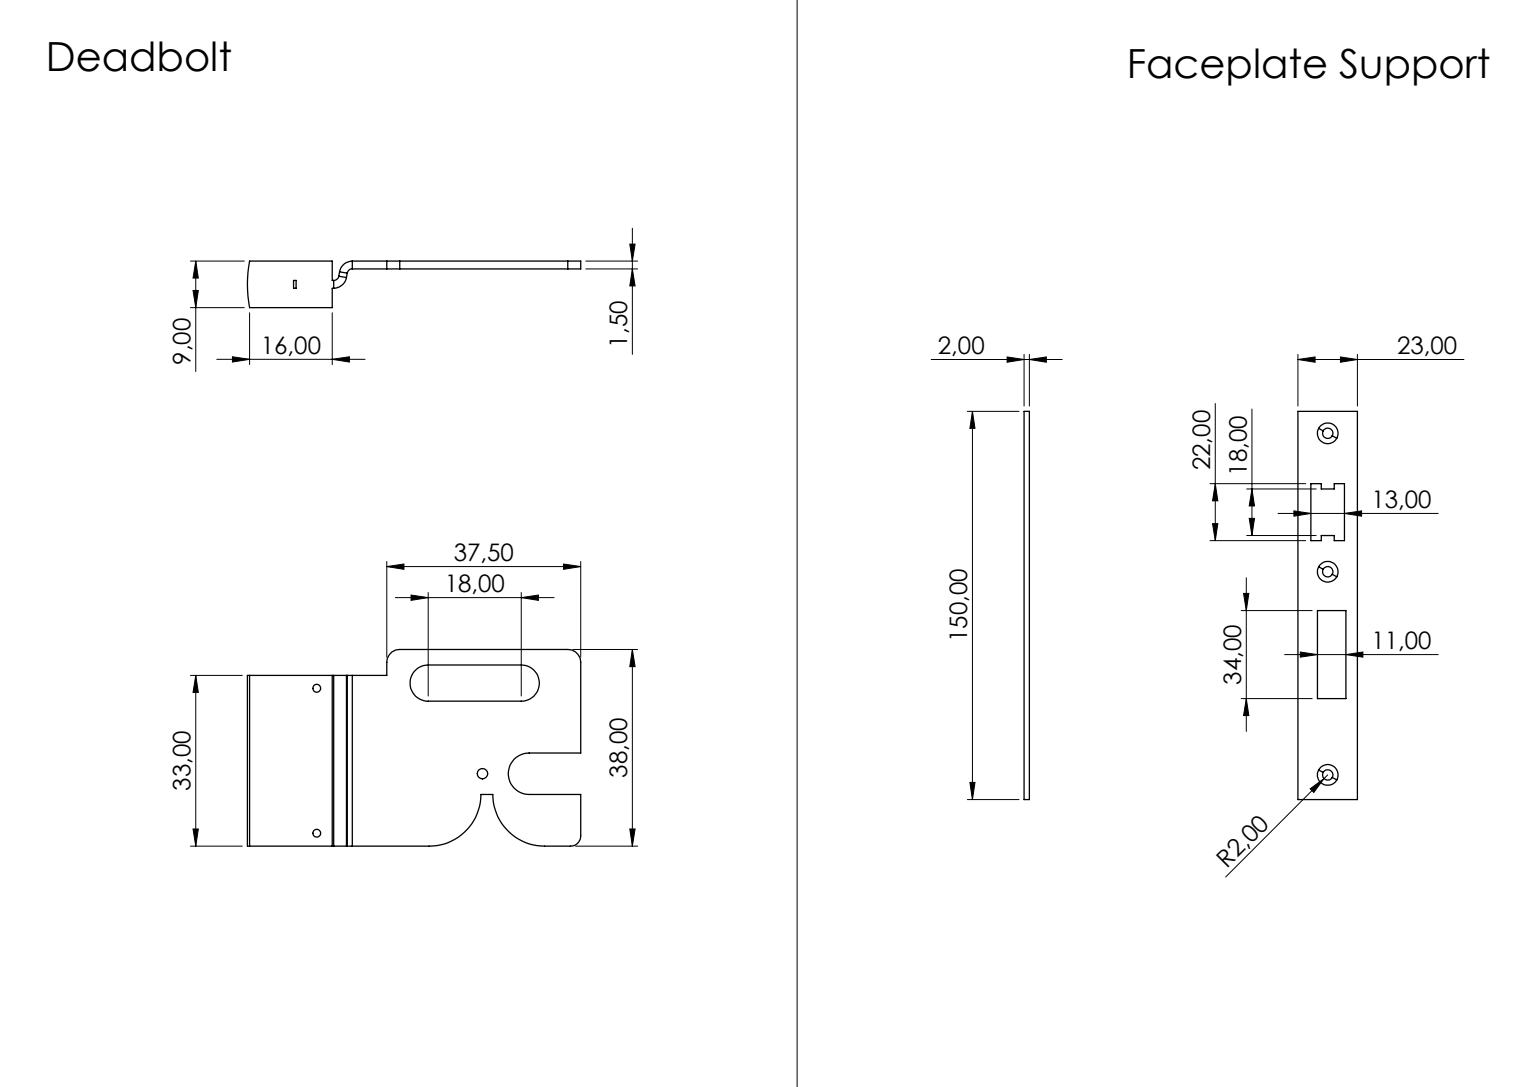
ISO-10303-21;
HEADER;
FILE_DESCRIPTION (('STEP AP214'),
    '1' );
FILE_NAME ('Faceplate Support.step',
    '2026-10-06T13:23:30',
    ( '' ),
    ( '' ),
    'SwSTEP 2.0',
    'SolidWorks 2020',
    '' );
FILE_SCHEMA (( 'AUTOMOTIVE_DESIGN' ));
ENDSEC;

DATA;
#73=VERTEX_POINT ( 'NONE', #5299 ) ;
#76=VERTEX_POINT ( 'NONE', #12547 ) ;
#94=VECTOR ( 'NONE', #6253, 1000.000000000000000 ) ;
#132=DIRECTION ( 'NONE',  ( 1.000000000000000000, 0.000000000000000000, 0.000000000000000000 ) ) ;
#135=DIRECTION ( 'NONE',  ( 1.000000000000000000, 2.602084704489999637E-17, 0.000000000000000000 ) ) ;
#145=FACE_BOUND ( 'NONE', #10019, .T. ) ;
#180=CARTESIAN_POINT ( 'NONE',  ( -33.42928932190000069, 66.02782287919998794, -146.7500980969999773 ) ) ;
#183=EDGE_LOOP ( 'NONE', ( #12514, #3187, #13299, #6261 ) ) ;
#184=EDGE_LOOP ( 'NONE', ( #18556, #23230 ) ) ;
#210=ADVANCED_FACE ( 'NONE', ( #13249 ), #13024, .F. ) ;
#292=LINE ( 'NONE', #7531, #4006 ) ;
#309=EDGE_LOOP ( 'NONE', ( #20160, #3924, #21001, #22212 ) ) ;
#317=CONICAL_SURFACE ( 'NONE', #15128, 1.999999999999992450, 0.7853981633970000820 ) ;
#385=FILL_AREA_STYLE_COLOUR ( '', #1433 ) ;
#392=LINE ( 'NONE', #16802, #3859 ) ;
#419=EDGE_LOOP ( 'NONE', ( #6689, #18751, #11885, #12680 ) ) ;
#431=ORIENTED_EDGE ( 'NONE', *, *, #17551, .T. ) ;
#453=ORIENTED_EDGE ( 'NONE', *, *, #12083, .T. ) ;
#485=PRESENTATION_STYLE_ASSIGNMENT (( #16769 ) ) ;
#517=DIRECTION ( 'NONE',  ( 0.000000000000000000, 0.000000000000000000, 1.000000000000000000 ) ) ;
#555=DIRECTION ( 'NONE',  ( -1.000000000000000000, 0.000000000000000000, 1.701177084980000217E-20 ) ) ;
#577=DIRECTION ( 'NONE',  ( 0.000000000000000000, -1.000000000000000000, 0.000000000000000000 ) ) ;
#623=PLANE ( 'NONE',  #6012 ) ;
#626=CARTESIAN_POINT ( 'NONE',  ( -32.50000000000000000, 27.00000000000000000, -141.5552959529999839 ) ) ;
#725=DIRECTION ( 'NONE',  ( 0.000000000000000000, 1.000000000000000000, 0.000000000000000000 ) ) ;
#777=VERTEX_POINT ( 'NONE', #13933 ) ;
#800=ORIENTED_EDGE ( 'NONE', *, *, #6653, .T. ) ;
#823=VECTOR ( 'NONE', #20074, 1000.000000000000000 ) ;
#843=CARTESIAN_POINT ( 'NONE',  ( -34.50000000000000000, -35.00000000000000000, -151.0552959529999839 ) ) ;
#845=VECTOR ( 'NONE', #2349, 1000.000000000000000 ) ;
#924=PLANE ( 'NONE',  #10610 ) ;
#925=CARTESIAN_POINT ( 'NONE',  ( -32.50000000000000000, 76.00000000000000000, -132.5552959530000123 ) ) ;
#927=CARTESIAN_POINT ( 'NONE',  ( -33.50000000000000000, -35.00000000000000000, -151.0552959529999839 ) ) ;
#941=VERTEX_POINT ( 'NONE', #11143 ) ;
#947=VERTEX_POINT ( 'NONE', #8804 ) ;
#969=DIRECTION ( 'NONE',  ( -1.000000000000000000, -2.602084704489999637E-17, 1.701177084830000066E-20 ) ) ;
#971=LINE ( 'NONE', #21197, #17113 ) ;
#1010=VECTOR ( 'NONE', #18945, 1000.000000000000000 ) ;
#1022=FACE_OUTER_BOUND ( 'NONE', #1478, .T. ) ;
#1026=LINE ( 'NONE', #6599, #12411 ) ;
#1069=VERTEX_POINT ( 'NONE', #925 ) ;
#1108=FACE_OUTER_BOUND ( 'NONE', #16737, .T. ) ;
#1156=VECTOR ( 'NONE', #20344, 1000.000000000000000 ) ;
#1161=DIRECTION ( 'NONE',  ( 1.000000000000000000, 0.000000000000000000, 0.000000000000000000 ) ) ;
#1195=DIRECTION ( 'NONE',  ( 1.000000000000000000, 2.004714280773594901E-17, -1.095180403012019938E-17 ) ) ;
#1238=AXIS2_PLACEMENT_3D ( 'NONE', #1926, #9145, #135 ) ;
#1262=DIRECTION ( 'NONE',  ( 0.000000000000000000, 0.000000000000000000, 1.000000000000000000 ) ) ;
#1350=LINE ( 'NONE', #10594, #19286 ) ;
#1398=EDGE_CURVE ( 'NONE', #23370, #2980, #10145, .T. ) ;
#1419=EDGE_CURVE ( 'NONE', #22886, #9252, #5700, .T. ) ;
#1422=VERTEX_POINT ( 'NONE', #4812 ) ;
#1433=COLOUR_RGB ( '', 0.31764706, 0.68627451, 0.89019608) ;
#1467=ADVANCED_FACE ( 'NONE', ( #15641 ), #8127, .F. ) ;
#1478=EDGE_LOOP ( 'NONE', ( #5603, #15343, #800, #15418 ) ) ;
#1527=VECTOR ( 'NONE', #2984, 1000.000000000000000 ) ;
#1629=PRODUCT ( 'Faceplate Support', 'Faceplate Support', '', ( #5675 ) ) ;
#1638=EDGE_LOOP ( 'NONE', ( #18762, #8978 ) ) ;
#1718=EDGE_CURVE ( 'NONE', #3899, #19035, #971, .T. ) ;
#1720=( LENGTH_UNIT ( ) NAMED_UNIT ( * ) SI_UNIT ( .MILLI., .METRE. ) );
#1770=EDGE_CURVE ( 'NONE', #4685, #18991, #9262, .T. ) ;
#1772=ORIENTED_EDGE ( 'NONE', *, *, #22316, .F. ) ;
#1774=ORIENTED_EDGE ( 'NONE', *, *, #4121, .F. ) ;
#1780=AXIS2_PLACEMENT_3D ( 'NONE', #5327, #3659, #9112 ) ;
#1819=ORIENTED_EDGE ( 'NONE', *, *, #16781, .T. ) ;
#1849=LINE ( 'NONE', #20040, #1010 ) ;
#1926=CARTESIAN_POINT ( 'NONE',  ( -32.50000000000000000, 48.00000000000000000, -146.5552959529999839 ) ) ;
#1931=DIRECTION ( 'NONE',  ( 0.000000000000000000, 1.000000000000000000, 0.000000000000000000 ) ) ;
#1948=LINE ( 'NONE', #3834, #4457 ) ;
#1951=DIRECTION ( 'NONE',  ( 1.000000000000000000, 2.004714280773594901E-17, -1.095180403012019938E-17 ) ) ;
#1984=ORIENTED_EDGE ( 'NONE', *, *, #6937, .F. ) ;
#2041=FACE_OUTER_BOUND ( 'NONE', #13396, .T. ) ;
#2052=CARTESIAN_POINT ( 'NONE',  ( -32.50000000000000000, 14.00000000000000000, -144.0552959529999839 ) ) ;
#2076=ORIENTED_EDGE ( 'NONE', *, *, #19643, .T. ) ;
#2094=ORIENTED_EDGE ( 'NONE', *, *, #16952, .F. ) ;
#2109=EDGE_CURVE ( 'NONE', #16248, #22948, #20352, .T. ) ;
#2111=VERTEX_POINT ( 'NONE', #11280 ) ;
#2132=ORIENTED_EDGE ( 'NONE', *, *, #13601, .T. ) ;
#2147=CARTESIAN_POINT ( 'NONE',  ( -34.50000000000000000, -1.000000000000000000, -145.5552959529999839 ) ) ;
#2158=DIRECTION ( 'NONE',  ( -1.000000000000000000, 0.000000000000000000, 0.000000000000000000 ) ) ;
#2182=PLANE ( 'NONE',  #20224 ) ;
#2191=EDGE_CURVE ( 'NONE', #4452, #11004, #2968, .T. ) ;
#2227=LINE ( 'NONE', #7560, #3466 ) ;
#2235=ORIENTED_EDGE ( 'NONE', *, *, #2191, .T. ) ;
#2272=FILL_AREA_STYLE_COLOUR ( '', #5063 ) ;
#2282=CARTESIAN_POINT ( 'NONE',  ( -32.50000000000000000, 48.00000000000000000, -139.5552959529999839 ) ) ;
#2311=VECTOR ( 'NONE', #4811, 1000.000000000000000 ) ;
#2349=DIRECTION ( 'NONE',  ( 0.000000000000000000, 0.000000000000000000, -1.000000000000000000 ) ) ;
#2386=CARTESIAN_POINT ( 'NONE',  ( -33.50000000000000000, 28.00000000000000000, -141.5552959529999839 ) ) ;
#2403=CARTESIAN_POINT ( 'NONE',  ( -32.50000000000000000, -1.000000000000000000, -151.0552959529999839 ) ) ;
#2432=EDGE_CURVE ( 'NONE', #18991, #13154, #12548, .T. ) ;
#2445=ORIENTED_EDGE ( 'NONE', *, *, #3029, .F. ) ;
#2460=PLANE ( 'NONE',  #7430 ) ;
#2478=DIRECTION ( 'NONE',  ( 0.000000000000000000, 1.000000000000000000, 0.000000000000000000 ) ) ;
#2576=CARTESIAN_POINT ( 'NONE',  ( -34.50000000000000000, -64.50000000000000000, -144.0552959529999839 ) ) ;
#2654=VECTOR ( 'NONE', #22857, 1000.000000000000000 ) ;
#2688=VECTOR ( 'NONE', #6527, 1000.000000000000000 ) ;
#2728=LINE ( 'NONE', #2835, #13984 ) ;
#2789=VERTEX_POINT ( 'NONE', #3495 ) ;
#2796=CARTESIAN_POINT ( 'NONE',  ( -32.50000000000000000, 48.00000000000000000, -148.5552959529999839 ) ) ;
#2797=DIRECTION ( 'NONE',  ( 1.000000000000000000, 2.602084704489999637E-17, -1.701177084830000066E-20 ) ) ;
#2835=CARTESIAN_POINT ( 'NONE',  ( -33.42928932190000069, 15.47217712079999963, -141.3604938089999905 ) ) ;
#2925=EDGE_LOOP ( 'NONE', ( #21956, #13989, #16727, #2445 ) ) ;
#2940=DIRECTION ( 'NONE',  ( 1.000000000000000000, 2.602084704489999637E-17, 0.000000000000000000 ) ) ;
#2955=CARTESIAN_POINT ( 'NONE',  ( -32.50000000000000000, -35.00000000000000000, -145.5552959529999839 ) ) ;
#2968=LINE ( 'NONE', #15450, #2688 ) ;
#2974=CARTESIAN_POINT ( 'NONE',  ( -34.50000000000000000, 67.50000000000000000, -144.0552959529999839 ) ) ;
#2980=VERTEX_POINT ( 'NONE', #4420 ) ;
#2984=DIRECTION ( 'NONE',  ( 0.000000000000000000, 1.000000000000000000, 0.000000000000000000 ) ) ;
#3029=EDGE_CURVE ( 'NONE', #1422, #22304, #7634, .T. ) ;
#3073=DIRECTION ( 'NONE',  ( 0.000000000000000000, 1.000000000000000000, 0.000000000000000000 ) ) ;
#3106=DIRECTION ( 'NONE',  ( 0.000000000000000000, 1.000000000000000000, 0.000000000000000000 ) ) ;
#3182=ORIENTED_EDGE ( 'NONE', *, *, #7620, .T. ) ;
#3187=ORIENTED_EDGE ( 'NONE', *, *, #20709, .F. ) ;
#3241=CARTESIAN_POINT ( 'NONE',  ( -32.50000000000000000, 48.00000000000000000, -146.5552959529999839 ) ) ;
#3284=VERTEX_POINT ( 'NONE', #20004 ) ;
#3338=VECTOR ( 'NONE', #7879, 1000.000000000000000 ) ;
#3382=DIRECTION ( 'NONE',  ( 0.000000000000000000, 1.000000000000000000, 0.000000000000000000 ) ) ;
#3388=ORIENTED_EDGE ( 'NONE', *, *, #3978, .T. ) ;
#3415=VECTOR ( 'NONE', #7837, 1000.000000000000000 ) ;
#3440=EDGE_CURVE ( 'NONE', #7907, #16321, #14757, .T. ) ;
#3466=VECTOR ( 'NONE', #22093, 1000.000000000000000 ) ;
#3482=DIRECTION ( 'NONE',  ( 0.000000000000000000, -0.4794255386042033384, -0.8775825618903726477 ) ) ;
#3495=CARTESIAN_POINT ( 'NONE',  ( -32.50000000000000000, 26.00000000000000000, -137.5552959530000123 ) ) ;
#3509=LINE ( 'NONE', #23142, #12900 ) ;
#3521=ORIENTED_EDGE ( 'NONE', *, *, #20709, .T. ) ;
#3536=( GEOMETRIC_REPRESENTATION_CONTEXT ( 3 ) GLOBAL_UNCERTAINTY_ASSIGNED_CONTEXT ( ( #12778 ) ) GLOBAL_UNIT_ASSIGNED_CONTEXT ( ( #1720, #9723, #18552 ) ) REPRESENTATION_CONTEXT ( 'NONE', 'WORKASPACE' ) );
#3538=VECTOR ( 'NONE', #15894, 1000.000000000000000 ) ;
#3572=ORIENTED_EDGE ( 'NONE', *, *, #6653, .F. ) ;
#3575=ADVANCED_FACE ( 'NONE', ( #10329 ), #5296, .F. ) ;
#3632=VERTEX_POINT ( 'NONE', #19148 ) ;
#3659=DIRECTION ( 'NONE',  ( -2.602084704489999637E-17, 1.000000000000000000, 4.426606872070000353E-37 ) ) ;
#3787=ORIENTED_EDGE ( 'NONE', *, *, #2432, .F. ) ;
#3830=ADVANCED_FACE ( 'NONE', ( #17834 ), #14508, .F. ) ;
#3834=CARTESIAN_POINT ( 'NONE',  ( -33.42928932190000069, -65.97217712079999785, -146.7500980969999773 ) ) ;
#3859=VECTOR ( 'NONE', #9637, 1000.000000000000000 ) ;
#3899=VERTEX_POINT ( 'NONE', #6151 ) ;
#3924=ORIENTED_EDGE ( 'NONE', *, *, #1718, .F. ) ;
#3978=EDGE_CURVE ( 'NONE', #18478, #16896, #20329, .T. ) ;
#4006=VECTOR ( 'NONE', #16698, 1000.000000000000000 ) ;
#4064=SURFACE_STYLE_FILL_AREA ( #20368 ) ;
#4121=EDGE_CURVE ( 'NONE', #13431, #13154, #4479, .T. ) ;
#4154=LINE ( 'NONE', #2386, #15576 ) ;
#4173=EDGE_CURVE ( 'NONE', #14517, #5601, #12435, .T. ) ;
#4195=FACE_OUTER_BOUND ( 'NONE', #22129, .T. ) ;
#4198=VECTOR ( 'NONE', #18442, 1000.000000000000114 ) ;
#4258=ORIENTED_EDGE ( 'NONE', *, *, #13581, .T. ) ;
#4270=CARTESIAN_POINT ( 'NONE',  ( -34.50000000000000000, 14.95885107719999851, -142.3001308290000111 ) ) ;
#4302=ORIENTED_EDGE ( 'NONE', *, *, #18394, .F. ) ;
#4391=CARTESIAN_POINT ( 'NONE',  ( -33.50000000000000000, 26.00000000000000000, -141.5552959529999839 ) ) ;
#4395=CIRCLE ( 'NONE', #21512, 2.000000000000001776 ) ;
#4403=CARTESIAN_POINT ( 'NONE',  ( -34.50000000000000000, -63.54114892279999793, -142.3001308290000111 ) ) ;
#4406=VECTOR ( 'NONE', #12477, 1000.000000000000000 ) ;
#4420=CARTESIAN_POINT ( 'NONE',  ( -32.50000000000000000, 46.00000000000000000, -141.5552959529999839 ) ) ;
#4452=VERTEX_POINT ( 'NONE', #17633 ) ;
#4456=DIRECTION ( 'NONE',  ( 0.000000000000000000, -1.000000000000000000, 0.000000000000000000 ) ) ;
#4457=VECTOR ( 'NONE', #9281, 1000.000000000000114 ) ;
#4460=ADVANCED_FACE ( 'NONE', ( #1108 ), #8680, .F. ) ;
#4479=LINE ( 'NONE', #927, #9677 ) ;
#4503=ORIENTED_EDGE ( 'NONE', *, *, #14997, .F. ) ;
#4509=VECTOR ( 'NONE', #10927, 1000.000000000000000 ) ;
#4510=CARTESIAN_POINT ( 'NONE',  ( -34.50000000000000000, 14.00000000000000000, -144.0552959529999839 ) ) ;
#4517=FACE_OUTER_BOUND ( 'NONE', #13767, .T. ) ;
#4555=ORIENTED_EDGE ( 'NONE', *, *, #8683, .F. ) ;
#4583=ADVANCED_FACE ( 'NONE', ( #10819, #23455, #10709, #145, #17991, #16440 ), #7388, .F. ) ;
#4590=CARTESIAN_POINT ( 'NONE',  ( 0.000000000000000000, 0.000000000000000000, 0.000000000000000000 ) ) ;
#4597=VECTOR ( 'NONE', #5076, 1000.000000000000000 ) ;
#4651=SURFACE_STYLE_USAGE ( .BOTH. , #18575 ) ;
#4676=ORIENTED_EDGE ( 'NONE', *, *, #16789, .T. ) ;
#4685=VERTEX_POINT ( 'NONE', #2403 ) ;
#4717=CARTESIAN_POINT ( 'NONE',  ( -34.50000000000000000, 26.00000000000000000, -150.5552959529999839 ) ) ;
#4756=EDGE_CURVE ( 'NONE', #19035, #777, #18565, .T. ) ;
#4764=( NAMED_UNIT ( * ) PLANE_ANGLE_UNIT ( ) SI_UNIT ( $, .RADIAN. ) );
#4811=DIRECTION ( 'NONE',  ( 0.000000000000000000, 0.000000000000000000, 1.000000000000000000 ) ) ;
#4812=CARTESIAN_POINT ( 'NONE',  ( -34.50000000000000000, 76.00000000000000000, -155.5552959529999839 ) ) ;
#4883=AXIS2_PLACEMENT_3D ( 'NONE', #16546, #10583, #11063 ) ;
#4916=DIRECTION ( 'NONE',  ( 1.000000000000000000, 0.000000000000000000, -1.701177084980000217E-20 ) ) ;
#4999=DIRECTION ( 'NONE',  ( -1.000000000000000000, 0.000000000000000000, 0.000000000000000000 ) ) ;
#5025=AXIS2_PLACEMENT_3D ( 'NONE', #4590, #17084, #1161 ) ;
#5029=CARTESIAN_POINT ( 'NONE',  ( -34.50000000000000000, -74.00000000000000000, -144.0552959529999839 ) ) ;
#5063=COLOUR_RGB ( '', 0.31764706, 0.68627451, 0.89019608) ;
#5068=ORIENTED_EDGE ( 'NONE', *, *, #14997, .T. ) ;
#5069=CARTESIAN_POINT ( 'NONE',  ( -34.50000000000000000, 46.00000000000000000, -141.5552959529999839 ) ) ;
#5076=DIRECTION ( 'NONE',  ( 0.000000000000000000, 0.000000000000000000, -1.000000000000000000 ) ) ;
#5080=EDGE_CURVE ( 'NONE', #4452, #947, #21998, .T. ) ;
#5094=FACE_OUTER_BOUND ( 'NONE', #18289, .T. ) ;
#5102=ORIENTED_EDGE ( 'NONE', *, *, #6464, .F. ) ;
#5106=ADVANCED_FACE ( 'NONE', ( #15207 ), #20443, .F. ) ;
#5153=EDGE_CURVE ( 'NONE', #3899, #19799, #15081, .T. ) ;
#5159=PLANE ( 'NONE',  #10966 ) ;
#5164=CARTESIAN_POINT ( 'NONE',  ( -33.50000000000000000, -35.00000000000000000, -140.0552959529999839 ) ) ;
#5194=ORIENTED_EDGE ( 'NONE', *, *, #12324, .F. ) ;
#5196=VERTEX_POINT ( 'NONE', #11257 ) ;
#5296=CONICAL_SURFACE ( 'NONE', #21657, 1.999999999999992450, 0.7853981633970000820 ) ;
#5299=CARTESIAN_POINT ( 'NONE',  ( -32.50000000000000000, 28.00000000000000000, -146.5552959529999839 ) ) ;
#5327=CARTESIAN_POINT ( 'NONE',  ( -32.50000000000000000, -1.000000000000000000, -140.0552959529999839 ) ) ;
#5371=VECTOR ( 'NONE', #12516, 1000.000000000000000 ) ;
#5384=EDGE_LOOP ( 'NONE', ( #17697, #4555, #4258, #11350 ) ) ;
#5441=ADVANCED_FACE ( 'NONE', ( #21476, #8717, #10618, #8954, #9066, #19572 ), #5159, .T. ) ;
#5442=ORIENTED_EDGE ( 'NONE', *, *, #15525, .F. ) ;
#5446=FACE_OUTER_BOUND ( 'NONE', #8558, .T. ) ;
#5452=CARTESIAN_POINT ( 'NONE',  ( -32.50000000000000000, 26.00000000000000000, -141.5552959529999839 ) ) ;
#5524=LINE ( 'NONE', #5164, #10885 ) ;
#5550=LINE ( 'NONE', #12797, #8991 ) ;
#5601=VERTEX_POINT ( 'NONE', #16927 ) ;
#5603=ORIENTED_EDGE ( 'NONE', *, *, #20750, .T. ) ;
#5640=UNCERTAINTY_MEASURE_WITH_UNIT (LENGTH_MEASURE( 1.000000000000000082E-05 ), #7720, 'distance_accuracy_value', 'NONE');
#5675=PRODUCT_CONTEXT ( 'NONE', #7803, 'mechanical' ) ;
#5687=VERTEX_POINT ( 'NONE', #22527 ) ;
#5700=CIRCLE ( 'NONE', #9102, 4.000000000000001776 ) ;
#5761=EDGE_LOOP ( 'NONE', ( #15101, #4676, #431, #2094 ) ) ;
#5783=EDGE_LOOP ( 'NONE', ( #21758, #22903, #22426, #6984 ) ) ;
#5803=ORIENTED_EDGE ( 'NONE', *, *, #1770, .T. ) ;
#5808=ADVANCED_BREP_SHAPE_REPRESENTATION ( '', ( #19584, #5025 ), #3536 ) ;
#5844=FACE_OUTER_BOUND ( 'NONE', #5761, .T. ) ;
#5867=DIRECTION ( 'NONE',  ( 0.000000000000000000, 1.000000000000000000, 0.000000000000000000 ) ) ;
#5885=ORIENTED_EDGE ( 'NONE', *, *, #19180, .F. ) ;
#5888=CARTESIAN_POINT ( 'NONE',  ( -34.50000000000000000, 67.50000000000000000, -144.0552959529999839 ) ) ;
#5902=DIRECTION ( 'NONE',  ( 0.7071067811866730279, 0.3390050494208429743, 0.6205445805637129775 ) ) ;
#5922=ORIENTED_EDGE ( 'NONE', *, *, #16952, .T. ) ;
#5944=CARTESIAN_POINT ( 'NONE',  ( -33.50000000000000000, 26.00000000000000000, -137.5552959530000123 ) ) ;
#5956=DIRECTION ( 'NONE',  ( 1.000000000000000000, 0.000000000000000000, 0.000000000000000000 ) ) ;
#5967=MECHANICAL_DESIGN_GEOMETRIC_PRESENTATION_REPRESENTATION('',(#8996),#23098);
#5979=CIRCLE ( 'NONE', #11285, 2.000000000000001776 ) ;
#6012=AXIS2_PLACEMENT_3D ( 'NONE', #13338, #18814, #22271 ) ;
#6036=CARTESIAN_POINT ( 'NONE',  ( -32.50000000000000000, 26.00000000000000000, -148.5552959529999839 ) ) ;
#6061=SURFACE_SIDE_STYLE ('',( #9497 ) ) ;
#6089=FACE_OUTER_BOUND ( 'NONE', #309, .T. ) ;
#6151=CARTESIAN_POINT ( 'NONE',  ( -32.50000000000000000, 26.00000000000000000, -146.5552959529999839 ) ) ;
#6228=VERTEX_POINT ( 'NONE', #23524 ) ;
#6253=DIRECTION ( 'NONE',  ( 0.000000000000000000, 1.000000000000000000, 0.000000000000000000 ) ) ;
#6261=ORIENTED_EDGE ( 'NONE', *, *, #20022, .T. ) ;
#6296=ORIENTED_EDGE ( 'NONE', *, *, #1398, .F. ) ;
#6301=VERTEX_POINT ( 'NONE', #21511 ) ;
#6353=CARTESIAN_POINT ( 'NONE',  ( -32.50000000000000000, 26.00000000000000000, -146.5552959529999839 ) ) ;
#6367=ORIENTED_EDGE ( 'NONE', *, *, #21785, .T. ) ;
#6378=DIRECTION ( 'NONE',  ( -2.602084704489999637E-17, 1.000000000000000000, 4.426606872070000353E-37 ) ) ;
#6382=ORIENTED_EDGE ( 'NONE', *, *, #7070, .F. ) ;
#6418=ORIENTED_EDGE ( 'NONE', *, *, #16781, .F. ) ;
#6422=AXIS2_PLACEMENT_3D ( 'NONE', #15804, #1195, #13901 ) ;
#6451=VECTOR ( 'NONE', #16424, 1000.000000000000000 ) ;
#6462=LINE ( 'NONE', #13475, #21120 ) ;
#6464=EDGE_CURVE ( 'NONE', #22304, #1069, #5550, .T. ) ;
#6477=CARTESIAN_POINT ( 'NONE',  ( -32.50000000000000000, 46.00000000000000000, -144.0552959529999839 ) ) ;
#6527=DIRECTION ( 'NONE',  ( -1.000000000000000000, 0.000000000000000000, 0.000000000000000000 ) ) ;
#6551=CARTESIAN_POINT ( 'NONE',  ( -32.50000000000000000, 15.91770215440000236, -140.5449657050000098 ) ) ;
#6590=DIRECTION ( 'NONE',  ( 1.000000000000000000, 0.000000000000000000, -1.701177084980000217E-20 ) ) ;
#6596=CARTESIAN_POINT ( 'NONE',  ( -32.50000000000000000, 48.00000000000000000, -150.5552959529999839 ) ) ;
#6599=CARTESIAN_POINT ( 'NONE',  ( -33.50000000000000000, -74.00000000000000000, -155.5552959529999839 ) ) ;
#6645=FACE_OUTER_BOUND ( 'NONE', #10270, .T. ) ;
#6653=EDGE_CURVE ( 'NONE', #19799, #6863, #9304, .T. ) ;
#6660=LINE ( 'NONE', #9142, #4406 ) ;
#6677=ORIENTED_EDGE ( 'NONE', *, *, #11955, .F. ) ;
#6689=ORIENTED_EDGE ( 'NONE', *, *, #17328, .F. ) ;
#6704=FACE_OUTER_BOUND ( 'NONE', #183, .T. ) ;
#6780=VECTOR ( 'NONE', #2478, 1000.000000000000000 ) ;
#6828=EDGE_LOOP ( 'NONE', ( #18220, #6296, #16409, #20832, #3572, #20707, #7912, #1772, #20208, #19025, #13112, #9318 ) ) ;
#6863=VERTEX_POINT ( 'NONE', #13947 ) ;
#6864=LINE ( 'NONE', #14707, #823 ) ;
#6937=EDGE_CURVE ( 'NONE', #16896, #15538, #1350, .T. ) ;
#6950=DIRECTION ( 'NONE',  ( 0.000000000000000000, 4.426606872070000353E-37, -1.000000000000000000 ) ) ;
#6952=CARTESIAN_POINT ( 'NONE',  ( -32.50000000000000000, -64.50000000000000000, -144.0552959529999839 ) ) ;
#6957=EDGE_CURVE ( 'NONE', #22660, #16248, #5979, .T. ) ;
#6984=ORIENTED_EDGE ( 'NONE', *, *, #19180, .T. ) ;
#6994=VECTOR ( 'NONE', #517, 1000.000000000000000 ) ;
#7005=VERTEX_POINT ( 'NONE', #3241 ) ;
#7070=EDGE_CURVE ( 'NONE', #22660, #8011, #1948, .T. ) ;
#7071=DIRECTION ( 'NONE',  ( 1.000000000000000000, 2.602084704489999637E-17, -1.701177084830000066E-20 ) ) ;
#7108=EDGE_LOOP ( 'NONE', ( #4503, #13044 ) ) ;
#7173=AXIS2_PLACEMENT_3D ( 'NONE', #18657, #11150, #7698 ) ;
#7214=ORIENTED_EDGE ( 'NONE', *, *, #7611, .T. ) ;
#7265=CARTESIAN_POINT ( 'NONE',  ( -34.50000000000000000, 67.50000000000000000, -144.0552959529999839 ) ) ;
#7279=LINE ( 'NONE', #5029, #15550 ) ;
#7280=LINE ( 'NONE', #11069, #21136 ) ;
#7286=CLOSED_SHELL ( 'NONE', ( #12650, #210, #13498, #22757, #10675, #13149, #19430, #3575, #3830, #17172, #18109, #15420, #4460, #10265, #14194, #23208, #8585, #20543, #1467, #18250, #19870, #8935, #5106, #22782, #5441, #4583, #21049, #20400 ) ) ;
#7324=CARTESIAN_POINT ( 'NONE',  ( -34.50000000000000000, -18.00000000000000000, -151.0552959529999839 ) ) ;
#7373=DIRECTION ( 'NONE',  ( -1.701177084980000217E-20, -4.426606872460000157E-37, -1.000000000000000000 ) ) ;
#7374=CARTESIAN_POINT ( 'NONE',  ( -33.50000000000000000, 76.00000000000000000, -155.5552959529999839 ) ) ;
#7387=DIRECTION ( 'NONE',  ( 1.000000000000000000, 2.602084704489999637E-17, -1.701177084830000066E-20 ) ) ;
#7388=PLANE ( 'NONE',  #4883 ) ;
#7403=CARTESIAN_POINT ( 'NONE',  ( -34.50000000000000000, 47.00000000000000000, -146.5552959529999839 ) ) ;
#7430=AXIS2_PLACEMENT_3D ( 'NONE', #9569, #9792, #555 ) ;
#7462=CARTESIAN_POINT ( 'NONE',  ( -32.50000000000000000, -35.00000000000000000, -151.0552959529999839 ) ) ;
#7500=ORIENTED_EDGE ( 'NONE', *, *, #4756, .F. ) ;
#7531=CARTESIAN_POINT ( 'NONE',  ( -34.50000000000000000, 0.9999999999959999775, -132.5552959530000123 ) ) ;
#7553=VECTOR ( 'NONE', #18883, 1000.000000000000000 ) ;
#7560=CARTESIAN_POINT ( 'NONE',  ( -32.50000000000000000, -1.000000000000000000, -145.5552959529999839 ) ) ;
#7597=LINE ( 'NONE', #10805, #1156 ) ;
#7611=EDGE_CURVE ( 'NONE', #13431, #4685, #20176, .T. ) ;
#7613=EDGE_LOOP ( 'NONE', ( #15509, #21470, #21303, #15582 ) ) ;
#7620=EDGE_CURVE ( 'NONE', #6228, #22167, #16825, .T. ) ;
#7634=LINE ( 'NONE', #18821, #6994 ) ;
#7653=DIRECTION ( 'NONE',  ( 1.000000000000000000, 2.602084704489999637E-17, -1.701177084830000066E-20 ) ) ;
#7698=DIRECTION ( 'NONE',  ( 1.000000000000000000, 0.000000000000000000, -1.701177084980000217E-20 ) ) ;
#7720=( LENGTH_UNIT ( ) NAMED_UNIT ( * ) SI_UNIT ( .MILLI., .METRE. ) );
#7784=EDGE_CURVE ( 'NONE', #22167, #6301, #21973, .T. ) ;
#7803=APPLICATION_CONTEXT ( 'automotive_design' ) ;
#7824=ORIENTED_EDGE ( 'NONE', *, *, #2109, .T. ) ;
#7837=DIRECTION ( 'NONE',  ( 0.000000000000000000, 0.000000000000000000, 1.000000000000000000 ) ) ;
#7839=CARTESIAN_POINT ( 'NONE',  ( -34.50000000000000000, 68.45885107719999496, -142.3001308290000111 ) ) ;
#7879=DIRECTION ( 'NONE',  ( 0.000000000000000000, 1.000000000000000000, 0.000000000000000000 ) ) ;
#7907=VERTEX_POINT ( 'NONE', #11535 ) ;
#7912=ORIENTED_EDGE ( 'NONE', *, *, #13581, .F. ) ;
#8011=VERTEX_POINT ( 'NONE', #11896 ) ;
#8083=( GEOMETRIC_REPRESENTATION_CONTEXT ( 3 ) GLOBAL_UNCERTAINTY_ASSIGNED_CONTEXT ( ( #5640 ) ) GLOBAL_UNIT_ASSIGNED_CONTEXT ( ( #7720, #22246, #22362 ) ) REPRESENTATION_CONTEXT ( 'NONE', 'WORKASPACE' ) );
#8126=DIRECTION ( 'NONE',  ( 0.000000000000000000, -0.4794255386042052813, -0.8775825618903714265 ) ) ;
#8127=PLANE ( 'NONE',  #12536 ) ;
#8133=PLANE ( 'NONE',  #22404 ) ;
#8149=DIRECTION ( 'NONE',  ( 1.000000000000000000, 2.602084704489999637E-17, 0.000000000000000000 ) ) ;
#8152=EDGE_CURVE ( 'NONE', #16321, #2789, #22240, .T. ) ;
#8181=DIRECTION ( 'NONE',  ( 1.000000000000000000, 2.004714280773594901E-17, -1.095180403012019938E-17 ) ) ;
#8194=CARTESIAN_POINT ( 'NONE',  ( -33.50000000000000000, 48.00000000000000000, -141.5552959529999839 ) ) ;
#8199=EDGE_LOOP ( 'NONE', ( #19667, #19295 ) ) ;
#8210=EDGE_CURVE ( 'NONE', #23370, #16366, #7597, .T. ) ;
#8254=DIRECTION ( 'NONE',  ( 1.000000000000000000, 0.000000000000000000, 0.000000000000000000 ) ) ;
#8306=ORIENTED_EDGE ( 'NONE', *, *, #18711, .T. ) ;
#8320=EDGE_CURVE ( 'NONE', #777, #2111, #12958, .T. ) ;
#8327=CARTESIAN_POINT ( 'NONE',  ( -33.42928932190000069, 12.52782287920000037, -146.7500980969999773 ) ) ;
#8386=CARTESIAN_POINT ( 'NONE',  ( -34.50000000000000000, -1.000000000000000000, -151.0552959529999839 ) ) ;
#8408=EDGE_CURVE ( 'NONE', #16967, #2111, #4154, .T. ) ;
#8486=LINE ( 'NONE', #2796, #2311 ) ;
#8558=EDGE_LOOP ( 'NONE', ( #19732, #21493, #15774, #2235 ) ) ;
#8575=LINE ( 'NONE', #21339, #17716 ) ;
#8582=CARTESIAN_POINT ( 'NONE',  ( -32.50000000000000000, 26.00000000000000000, -139.5552959529999839 ) ) ;
#8585=ADVANCED_FACE ( 'NONE', ( #1022 ), #8133, .F. ) ;
#8594=ORIENTED_EDGE ( 'NONE', *, *, #19813, .F. ) ;
#8605=DIRECTION ( 'NONE',  ( 0.000000000000000000, 1.000000000000000000, 0.000000000000000000 ) ) ;
#8615=ORIENTED_EDGE ( 'NONE', *, *, #6957, .T. ) ;
#8680=PLANE ( 'NONE',  #16289 ) ;
#8683=EDGE_CURVE ( 'NONE', #73, #777, #3509, .T. ) ;
#8698=ORIENTED_EDGE ( 'NONE', *, *, #16627, .F. ) ;
#8717=FACE_BOUND ( 'NONE', #22780, .T. ) ;
#8730=ORIENTED_EDGE ( 'NONE', *, *, #17551, .F. ) ;
#8743=LINE ( 'NONE', #12319, #3538 ) ;
#8754=PRODUCT_DEFINITION ( 'UNKNOWN', '', #11884, #10159 ) ;
#8804=CARTESIAN_POINT ( 'NONE',  ( -32.50000000000000000, -35.00000000000000000, -140.0552959529999839 ) ) ;
#8807=EDGE_LOOP ( 'NONE', ( #1984, #17604, #4302, #15669, #14090, #7500, #8698, #16036, #12638, #11124, #12711, #20343 ) ) ;
#8812=PRODUCT_DEFINITION_SHAPE ( 'NONE', 'NONE',  #8754 ) ;
#8935=ADVANCED_FACE ( 'NONE', ( #5094 ), #16043, .F. ) ;
#8954=FACE_BOUND ( 'NONE', #184, .T. ) ;
#8976=CARTESIAN_POINT ( 'NONE',  ( -32.50000000000000000, 27.00000000000000000, -146.5552959529999839 ) ) ;
#8978=ORIENTED_EDGE ( 'NONE', *, *, #6957, .F. ) ;
#8991=VECTOR ( 'NONE', #14945, 1000.000000000000000 ) ;
#8996=STYLED_ITEM ( 'NONE', ( #17494 ), #19584 ) ;
#9012=LINE ( 'NONE', #19519, #15462 ) ;
#9066=FACE_BOUND ( 'NONE', #12387, .T. ) ;
#9086=DIRECTION ( 'NONE',  ( -1.000000000000000000, 0.000000000000000000, 0.000000000000000000 ) ) ;
#9102=AXIS2_PLACEMENT_3D ( 'NONE', #17659, #2797, #21119 ) ;
#9112=DIRECTION ( 'NONE',  ( 1.000000000000000000, 2.602084704489999637E-17, 0.000000000000000000 ) ) ;
#9117=DIRECTION ( 'NONE',  ( 0.000000000000000000, 4.426606872070000353E-37, -1.000000000000000000 ) ) ;
#9127=DIRECTION ( 'NONE',  ( 2.602084704489999637E-17, -1.000000000000000000, -4.426606872070000353E-37 ) ) ;
#9142=CARTESIAN_POINT ( 'NONE',  ( -34.50000000000000000, -35.00000000000000000, -145.5552959529999839 ) ) ;
#9145=DIRECTION ( 'NONE',  ( -2.602084704489999637E-17, 1.000000000000000000, 4.426606872070000353E-37 ) ) ;
#9158=AXIS2_PLACEMENT_3D ( 'NONE', #7265, #19769, #1931 ) ;
#9177=LINE ( 'NONE', #7403, #5371 ) ;
#9203=UNCERTAINTY_MEASURE_WITH_UNIT (LENGTH_MEASURE( 1.000000000000000082E-05 ), #21078, 'distance_accuracy_value', 'NONE');
#9252=VERTEX_POINT ( 'NONE', #16370 ) ;
#9262=LINE ( 'NONE', #12957, #11413 ) ;
#9263=CARTESIAN_POINT ( 'NONE',  ( -34.50000000000000000, 28.00000000000000000, -144.0552959529999839 ) ) ;
#9281=DIRECTION ( 'NONE',  ( 0.7071067811866730279, -0.3390050494208429743, -0.6205445805637129775 ) ) ;
#9287=PLANE ( 'NONE',  #15643 ) ;
#9295=VERTEX_POINT ( 'NONE', #5069 ) ;
#9304=LINE ( 'NONE', #18374, #21947 ) ;
#9318=ORIENTED_EDGE ( 'NONE', *, *, #3440, .F. ) ;
#9421=LINE ( 'NONE', #22181, #17288 ) ;
#9497=SURFACE_STYLE_FILL_AREA ( #22482 ) ;
#9507=CARTESIAN_POINT ( 'NONE',  ( -34.50000000000000000, 27.00000000000000000, -146.5552959529999839 ) ) ;
#9524=DIRECTION ( 'NONE',  ( 1.000000000000000000, 2.602084704489999637E-17, 0.000000000000000000 ) ) ;
#9545=CIRCLE ( 'NONE', #9158, 2.000000000000001776 ) ;
#9560=AXIS2_PLACEMENT_3D ( 'NONE', #17056, #22424, #12903 ) ;
#9569=CARTESIAN_POINT ( 'NONE',  ( -32.50000000000000000, -1.000000000000000000, -151.0552959529999839 ) ) ;
#9604=LINE ( 'NONE', #2147, #22328 ) ;
#9637=DIRECTION ( 'NONE',  ( 0.000000000000000000, 0.000000000000000000, 1.000000000000000000 ) ) ;
#9677=VECTOR ( 'NONE', #22684, 1000.000000000000000 ) ;
#9713=CARTESIAN_POINT ( 'NONE',  ( -32.50000000000000000, 28.00000000000000000, -141.5552959529999839 ) ) ;
#9723=( NAMED_UNIT ( * ) PLANE_ANGLE_UNIT ( ) SI_UNIT ( $, .RADIAN. ) );
#9731=EDGE_CURVE ( 'NONE', #3632, #16983, #18557, .T. ) ;
#9747=CARTESIAN_POINT ( 'NONE',  ( -32.50000000000000000, 48.00000000000000000, -146.5552959529999839 ) ) ;
#9758=DIRECTION ( 'NONE',  ( -1.000000000000000000, 0.000000000000000000, 0.000000000000000000 ) ) ;
#9792=DIRECTION ( 'NONE',  ( -1.701177084980000217E-20, -4.426606872460000157E-37, -1.000000000000000000 ) ) ;
#9818=CARTESIAN_POINT ( 'NONE',  ( -34.50000000000000000, -1.000000000000000000, -140.0552959529999839 ) ) ;
#9923=AXIS2_PLACEMENT_3D ( 'NONE', #17022, #11303, #18579 ) ;
#9938=FACE_OUTER_BOUND ( 'NONE', #419, .T. ) ;
#9965=VECTOR ( 'NONE', #10520, 1000.000000000000000 ) ;
#9975=ORIENTED_EDGE ( 'NONE', *, *, #18080, .F. ) ;
#10019=EDGE_LOOP ( 'NONE', ( #6418, #9975 ) ) ;
#10027=CARTESIAN_POINT ( 'NONE',  ( -34.50000000000000000, 27.00000000000000000, -141.5552959529999839 ) ) ;
#10035=CARTESIAN_POINT ( 'NONE',  ( -34.50000000000000000, 26.00000000000000000, -146.5552959529999839 ) ) ;
#10076=ORIENTED_EDGE ( 'NONE', *, *, #8408, .F. ) ;
#10085=ORIENTED_EDGE ( 'NONE', *, *, #22460, .F. ) ;
#10097=AXIS2_PLACEMENT_3D ( 'NONE', #10538, #23531, #10894 ) ;
#10099=CARTESIAN_POINT ( 'NONE',  ( -34.50000000000000000, -64.50000000000000000, -144.0552959529999839 ) ) ;
#10106=LINE ( 'NONE', #8327, #23503 ) ;
#10145=LINE ( 'NONE', #6477, #17095 ) ;
#10159=PRODUCT_DEFINITION_CONTEXT ( 'detailed design', #14809, 'design' ) ;
#10161=VECTOR ( 'NONE', #22295, 1000.000000000000114 ) ;
#10172=VERTEX_POINT ( 'NONE', #4717 ) ;
#10193=CARTESIAN_POINT ( 'NONE',  ( -33.50000000000000000, 48.00000000000000000, -150.5552959529999839 ) ) ;
#10265=ADVANCED_FACE ( 'NONE', ( #17207 ), #924, .F. ) ;
#10270=EDGE_LOOP ( 'NONE', ( #12457, #11238, #1819, #3521 ) ) ;
#10326=DIRECTION ( 'NONE',  ( 0.000000000000000000, -0.4794255386042052813, -0.8775825618903714265 ) ) ;
#10329=FACE_OUTER_BOUND ( 'NONE', #17115, .T. ) ;
#10365=DIRECTION ( 'NONE',  ( -1.000000000000000000, 0.000000000000000000, 0.000000000000000000 ) ) ;
#10372=LINE ( 'NONE', #8582, #845 ) ;
#10396=CARTESIAN_POINT ( 'NONE',  ( -34.50000000000000000, 14.00000000000000000, -144.0552959529999839 ) ) ;
#10433=ORIENTED_EDGE ( 'NONE', *, *, #3440, .T. ) ;
#10454=VECTOR ( 'NONE', #5956, 1000.000000000000000 ) ;
#10505=EDGE_CURVE ( 'NONE', #19799, #10172, #18624, .T. ) ;
#10513=LINE ( 'NONE', #19824, #13341 ) ;
#10520=DIRECTION ( 'NONE',  ( 0.000000000000000000, -1.000000000000000000, 0.000000000000000000 ) ) ;
#10521=CARTESIAN_POINT ( 'NONE',  ( -32.50000000000000000, -74.00000000000000000, -144.0552959529999839 ) ) ;
#10528=CARTESIAN_POINT ( 'NONE',  ( -32.50000000000000000, 67.50000000000000000, -144.0552959529999839 ) ) ;
#10538=CARTESIAN_POINT ( 'NONE',  ( -34.50000000000000000, 14.00000000000000000, -144.0552959529999839 ) ) ;
#10542=ORIENTED_EDGE ( 'NONE', *, *, #16018, .F. ) ;
#10583=DIRECTION ( 'NONE',  ( 1.000000000000000000, 2.602084704489999637E-17, -1.701177084830000066E-20 ) ) ;
#10591=EDGE_CURVE ( 'NONE', #6863, #7005, #8486, .T. ) ;
#10594=CARTESIAN_POINT ( 'NONE',  ( -34.50000000000000000, 48.00000000000000000, -139.5552959529999839 ) ) ;
#10596=EDGE_LOOP ( 'NONE', ( #10777, #5885, #12308, #18566 ) ) ;
#10610=AXIS2_PLACEMENT_3D ( 'NONE', #22808, #12080, #8149 ) ;
#10618=FACE_BOUND ( 'NONE', #7108, .T. ) ;
#10675=ADVANCED_FACE ( 'NONE', ( #6704 ), #11373, .F. ) ;
#10709=FACE_BOUND ( 'NONE', #8199, .T. ) ;
#10741=DIRECTION ( 'NONE',  ( -1.000000000000000000, 0.000000000000000000, 0.000000000000000000 ) ) ;
#10777=ORIENTED_EDGE ( 'NONE', *, *, #17549, .T. ) ;
#10805=CARTESIAN_POINT ( 'NONE',  ( -33.50000000000000000, 46.00000000000000000, -146.5552959529999839 ) ) ;
#10819=FACE_BOUND ( 'NONE', #8807, .T. ) ;
#10836=CARTESIAN_POINT ( 'NONE',  ( -34.50000000000000000, -65.45885107719999496, -145.8104610769999852 ) ) ;
#10854=DIRECTION ( 'NONE',  ( 1.000000000000000000, 2.602084704489999637E-17, -1.701177084830000066E-20 ) ) ;
#10885=VECTOR ( 'NONE', #23493, 1000.000000000000000 ) ;
#10894=DIRECTION ( 'NONE',  ( 0.000000000000000000, 1.000000000000000000, 0.000000000000000000 ) ) ;
#10927=DIRECTION ( 'NONE',  ( 0.000000000000000000, -1.000000000000000000, 0.000000000000000000 ) ) ;
#10946=VECTOR ( 'NONE', #725, 1000.000000000000000 ) ;
#10966=AXIS2_PLACEMENT_3D ( 'NONE', #23487, #10854, #14095 ) ;
#10989=ORIENTED_EDGE ( 'NONE', *, *, #23347, .F. ) ;
#11004=VERTEX_POINT ( 'NONE', #9818 ) ;
#11063=DIRECTION ( 'NONE',  ( -2.602084704489999637E-17, 1.000000000000000000, 0.000000000000000000 ) ) ;
#11069=CARTESIAN_POINT ( 'NONE',  ( -32.50000000000000000, 0.9999999999959999775, -132.5552959530000123 ) ) ;
#11112=DIRECTION ( 'NONE',  ( 0.000000000000000000, -1.000000000000000000, 0.000000000000000000 ) ) ;
#11124=ORIENTED_EDGE ( 'NONE', *, *, #11837, .F. ) ;
#11143=CARTESIAN_POINT ( 'NONE',  ( -34.50000000000000000, 13.04114892279999971, -145.8104610769999852 ) ) ;
#11150=DIRECTION ( 'NONE',  ( 1.701177084980000217E-20, 4.426606872460000157E-37, 1.000000000000000000 ) ) ;
#11187=CARTESIAN_POINT ( 'NONE',  ( -32.50000000000000000, 67.50000000000000000, -144.0552959529999839 ) ) ;
#11191=VECTOR ( 'NONE', #17558, 1000.000000000000000 ) ;
#11238=ORIENTED_EDGE ( 'NONE', *, *, #20022, .F. ) ;
#11257=CARTESIAN_POINT ( 'NONE',  ( -34.50000000000000000, 48.00000000000000000, -150.5552959529999839 ) ) ;
#11280=CARTESIAN_POINT ( 'NONE',  ( -34.50000000000000000, 28.00000000000000000, -141.5552959529999839 ) ) ;
#11285=AXIS2_PLACEMENT_3D ( 'NONE', #23350, #15848, #14302 ) ;
#11301=AXIS2_PLACEMENT_3D ( 'NONE', #11187, #11302, #20147 ) ;
#11302=DIRECTION ( 'NONE',  ( 1.000000000000000000, 2.602084704489999637E-17, -1.701177084830000066E-20 ) ) ;
#11303=DIRECTION ( 'NONE',  ( 1.701177084980000217E-20, 4.426606872460000157E-37, 1.000000000000000000 ) ) ;
#11329=VECTOR ( 'NONE', #577, 1000.000000000000000 ) ;
#11332=ORIENTED_EDGE ( 'NONE', *, *, #17549, .F. ) ;
#11350=ORIENTED_EDGE ( 'NONE', *, *, #1718, .T. ) ;
#11356=ORIENTED_EDGE ( 'NONE', *, *, #21121, .T. ) ;
#11373=CONICAL_SURFACE ( 'NONE', #12150, 1.999999999999995115, 0.7853981633970000820 ) ;
#11384=EDGE_CURVE ( 'NONE', #2111, #16983, #13491, .T. ) ;
#11387=ORIENTED_EDGE ( 'NONE', *, *, #10591, .T. ) ;
#11394=PLANE ( 'NONE',  #1238 ) ;
#11401=CARTESIAN_POINT ( 'NONE',  ( -33.42928932190000069, -63.02782287919998794, -141.3604938089999905 ) ) ;
#11413=VECTOR ( 'NONE', #12606, 1000.000000000000000 ) ;
#11422=CARTESIAN_POINT ( 'NONE',  ( -33.50000000000000000, -74.00000000000000000, -132.5552959530000123 ) ) ;
#11433=DIRECTION ( 'NONE',  ( 0.000000000000000000, 4.426606872070000353E-37, -1.000000000000000000 ) ) ;
#11492=CARTESIAN_POINT ( 'NONE',  ( -32.50000000000000000, -74.00000000000000000, -132.5552959530000123 ) ) ;
#11502=FACE_OUTER_BOUND ( 'NONE', #19955, .T. ) ;
#11526=CARTESIAN_POINT ( 'NONE',  ( -34.50000000000000000, 26.00000000000000000, -137.5552959530000123 ) ) ;
#11535=CARTESIAN_POINT ( 'NONE',  ( -32.50000000000000000, 48.00000000000000000, -141.5552959529999839 ) ) ;
#11591=CARTESIAN_POINT ( 'NONE',  ( -34.50000000000000000, -18.00000000000000000, -140.0552959529999839 ) ) ;
#11601=CARTESIAN_POINT ( 'NONE',  ( -34.50000000000000000, -74.00000000000000000, -155.5552959529999839 ) ) ;
#11625=CIRCLE ( 'NONE', #10097, 2.000000000000000000 ) ;
#11629=ORIENTED_EDGE ( 'NONE', *, *, #7620, .F. ) ;
#11657=DIRECTION ( 'NONE',  ( 0.000000000000000000, 1.000000000000000000, 0.000000000000000000 ) ) ;
#11678=CARTESIAN_POINT ( 'NONE',  ( -32.50000000000000000, 28.00000000000000000, -141.5552959529999839 ) ) ;
#11729=AXIS2_PLACEMENT_3D ( 'NONE', #10528, #15902, #3073 ) ;
#11731=ORIENTED_EDGE ( 'NONE', *, *, #16454, .F. ) ;
#11837=EDGE_CURVE ( 'NONE', #16366, #18905, #9177, .T. ) ;
#11862=ORIENTED_EDGE ( 'NONE', *, *, #16898, .T. ) ;
#11880=ORIENTED_EDGE ( 'NONE', *, *, #6464, .T. ) ;
#11884=PRODUCT_DEFINITION_FORMATION_WITH_SPECIFIED_SOURCE ( 'ANY', '', #1629, .NOT_KNOWN. ) ;
#11885=ORIENTED_EDGE ( 'NONE', *, *, #19045, .T. ) ;
#11896=CARTESIAN_POINT ( 'NONE',  ( -32.50000000000000000, -66.41770215440000413, -147.5656262009999864 ) ) ;
#11955=EDGE_CURVE ( 'NONE', #3284, #1069, #392, .T. ) ;
#11956=ORIENTED_EDGE ( 'NONE', *, *, #12977, .F. ) ;
#12080=DIRECTION ( 'NONE',  ( -2.602084704489999637E-17, 1.000000000000000000, 4.426606872070000353E-37 ) ) ;
#12082=PLANE ( 'NONE',  #12250 ) ;
#12083=EDGE_CURVE ( 'NONE', #6228, #14075, #9545, .T. ) ;
#12097=DIRECTION ( 'NONE',  ( 0.000000000000000000, 0.000000000000000000, -1.000000000000000000 ) ) ;
#12116=CIRCLE ( 'NONE', #11729, 4.000000000000003553 ) ;
#12150=AXIS2_PLACEMENT_3D ( 'NONE', #19199, #17062, #8126 ) ;
#12210=EDGE_LOOP ( 'NONE', ( #14021, #1774, #7214, #5803 ) ) ;
#12250=AXIS2_PLACEMENT_3D ( 'NONE', #11601, #6378, #2940 ) ;
#12278=CARTESIAN_POINT ( 'NONE',  ( -32.50000000000000000, -35.00000000000000000, -140.0552959529999839 ) ) ;
#12308=ORIENTED_EDGE ( 'NONE', *, *, #19990, .T. ) ;
#12319=CARTESIAN_POINT ( 'NONE',  ( -32.50000000000000000, 47.00000000000000000, -146.5552959529999839 ) ) ;
#12324=EDGE_CURVE ( 'NONE', #2980, #9295, #10513, .T. ) ;
#12351=DIRECTION ( 'NONE',  ( 0.000000000000000000, -1.000000000000000000, 0.000000000000000000 ) ) ;
#12387=EDGE_LOOP ( 'NONE', ( #22746, #5442 ) ) ;
#12411=VECTOR ( 'NONE', #8254, 1000.000000000000000 ) ;
#12435=LINE ( 'NONE', #10521, #4597 ) ;
#12457=ORIENTED_EDGE ( 'NONE', *, *, #14028, .T. ) ;
#12470=EDGE_LOOP ( 'NONE', ( #5102, #11862, #17850, #18148 ) ) ;
#12477=DIRECTION ( 'NONE',  ( 0.000000000000000000, 0.000000000000000000, 1.000000000000000000 ) ) ;
#12514=ORIENTED_EDGE ( 'NONE', *, *, #1419, .T. ) ;
#12516=DIRECTION ( 'NONE',  ( 0.000000000000000000, 1.000000000000000000, 0.000000000000000000 ) ) ;
#12536=AXIS2_PLACEMENT_3D ( 'NONE', #6353, #22905, #6590 ) ;
#12547=CARTESIAN_POINT ( 'NONE',  ( -34.50000000000000000, -35.00000000000000000, -140.0552959529999839 ) ) ;
#12548=LINE ( 'NONE', #7324, #18379 ) ;
#12553=LINE ( 'NONE', #8976, #9965 ) ;
#12606=DIRECTION ( 'NONE',  ( -1.000000000000000000, 0.000000000000000000, 0.000000000000000000 ) ) ;
#12609=LINE ( 'NONE', #14400, #4509 ) ;
#12638=ORIENTED_EDGE ( 'NONE', *, *, #21730, .F. ) ;
#12650=ADVANCED_FACE ( 'NONE', ( #4195 ), #2182, .F. ) ;
#12652=EDGE_CURVE ( 'NONE', #3632, #16967, #15370, .T. ) ;
#12661=VERTEX_POINT ( 'NONE', #17436 ) ;
#12662=DIRECTION ( 'NONE',  ( 0.000000000000000000, 1.000000000000000000, 0.000000000000000000 ) ) ;
#12680=ORIENTED_EDGE ( 'NONE', *, *, #4173, .F. ) ;
#12711=ORIENTED_EDGE ( 'NONE', *, *, #22479, .F. ) ;
#12730=VECTOR ( 'NONE', #4999, 1000.000000000000000 ) ;
#12778=UNCERTAINTY_MEASURE_WITH_UNIT (LENGTH_MEASURE( 1.000000000000000082E-05 ), #1720, 'distance_accuracy_value', 'NONE');
#12797=CARTESIAN_POINT ( 'NONE',  ( -33.50000000000000000, 76.00000000000000000, -132.5552959530000123 ) ) ;
#12847=ORIENTED_EDGE ( 'NONE', *, *, #19990, .F. ) ;
#12895=CARTESIAN_POINT ( 'NONE',  ( -32.50000000000000000, -18.00000000000000000, -151.0552959529999839 ) ) ;
#12900=VECTOR ( 'NONE', #10741, 1000.000000000000000 ) ;
#12903=DIRECTION ( 'NONE',  ( -1.000000000000000000, 0.000000000000000000, 1.701177084980000217E-20 ) ) ;
#12957=CARTESIAN_POINT ( 'NONE',  ( -33.50000000000000000, -1.000000000000000000, -151.0552959529999839 ) ) ;
#12958=LINE ( 'NONE', #9263, #6451 ) ;
#12977=EDGE_CURVE ( 'NONE', #2789, #18478, #22253, .T. ) ;
#13024=PLANE ( 'NONE',  #9560 ) ;
#13028=CARTESIAN_POINT ( 'NONE',  ( -33.50000000000000000, 26.00000000000000000, -150.5552959529999839 ) ) ;
#13037=STYLED_ITEM ( 'NONE', ( #485 ), #5808 ) ;
#13044=ORIENTED_EDGE ( 'NONE', *, *, #7784, .F. ) ;
#13112=ORIENTED_EDGE ( 'NONE', *, *, #8152, .F. ) ;
#13124=CARTESIAN_POINT ( 'NONE',  ( -32.50000000000000000, -64.50000000000000000, -144.0552959529999839 ) ) ;
#13136=AXIS2_PLACEMENT_3D ( 'NONE', #6952, #7071, #3382 ) ;
#13149=ADVANCED_FACE ( 'NONE', ( #6645 ), #20625, .F. ) ;
#13154=VERTEX_POINT ( 'NONE', #843 ) ;
#13201=VECTOR ( 'NONE', #12097, 1000.000000000000000 ) ;
#13237=AXIS2_PLACEMENT_3D ( 'NONE', #2052, #7387, #14293 ) ;
#13249=FACE_OUTER_BOUND ( 'NONE', #12470, .T. ) ;
#13260=FACE_OUTER_BOUND ( 'NONE', #12210, .T. ) ;
#13299=ORIENTED_EDGE ( 'NONE', *, *, #18080, .T. ) ;
#13338=CARTESIAN_POINT ( 'NONE',  ( -32.50000000000000000, 26.00000000000000000, -141.5552959529999839 ) ) ;
#13341=VECTOR ( 'NONE', #9086, 1000.000000000000000 ) ;
#13344=DIRECTION ( 'NONE',  ( 2.602084704489999637E-17, -1.000000000000000000, -4.426606872070000353E-37 ) ) ;
#13359=VECTOR ( 'NONE', #11657, 1000.000000000000000 ) ;
#13396=EDGE_LOOP ( 'NONE', ( #21796, #10989, #11387, #14946 ) ) ;
#13431=VERTEX_POINT ( 'NONE', #7462 ) ;
#13475=CARTESIAN_POINT ( 'NONE',  ( -32.50000000000000000, 0.9999999999959999775, -155.5552959529999839 ) ) ;
#13491=LINE ( 'NONE', #10027, #18647 ) ;
#13498=ADVANCED_FACE ( 'NONE', ( #9938 ), #12082, .F. ) ;
#13506=ORIENTED_EDGE ( 'NONE', *, *, #15168, .T. ) ;
#13561=EDGE_CURVE ( 'NONE', #7005, #23370, #8743, .T. ) ;
#13581=EDGE_CURVE ( 'NONE', #73, #3899, #12553, .T. ) ;
#13601=EDGE_CURVE ( 'NONE', #16321, #16896, #22632, .T. ) ;
#13691=DIRECTION ( 'NONE',  ( -1.000000000000000000, 0.000000000000000000, 0.000000000000000000 ) ) ;
#13720=VECTOR ( 'NONE', #15743, 1000.000000000000000 ) ;
#13757=ORIENTED_EDGE ( 'NONE', *, *, #16800, .T. ) ;
#13767=EDGE_LOOP ( 'NONE', ( #23497, #10542, #15755, #17709 ) ) ;
#13794=MECHANICAL_DESIGN_GEOMETRIC_PRESENTATION_REPRESENTATION('',(#13037),#8083);
#13804=DIRECTION ( 'NONE',  ( 1.701177084980000217E-20, 4.426606872460000157E-37, 1.000000000000000000 ) ) ;
#13858=DIRECTION ( 'NONE',  ( 2.602084704489999637E-17, -1.000000000000000000, -4.426606872070000353E-37 ) ) ;
#13890=CIRCLE ( 'NONE', #13136, 4.000000000000003553 ) ;
#13901=DIRECTION ( 'NONE',  ( 0.000000000000000000, -0.4794255386042033384, -0.8775825618903726477 ) ) ;
#13912=PLANE ( 'NONE',  #20491 ) ;
#13920=CARTESIAN_POINT ( 'NONE',  ( -34.50000000000000000, 48.00000000000000000, -148.5552959529999839 ) ) ;
#13933=CARTESIAN_POINT ( 'NONE',  ( -34.50000000000000000, 28.00000000000000000, -146.5552959529999839 ) ) ;
#13939=CARTESIAN_POINT ( 'NONE',  ( -32.50000000000000000, 28.00000000000000000, -141.5552959529999839 ) ) ;
#13947=CARTESIAN_POINT ( 'NONE',  ( -32.50000000000000000, 48.00000000000000000, -150.5552959529999839 ) ) ;
#13984=VECTOR ( 'NONE', #14491, 1000.000000000000114 ) ;
#13989=ORIENTED_EDGE ( 'NONE', *, *, #21337, .F. ) ;
#14021=ORIENTED_EDGE ( 'NONE', *, *, #2432, .T. ) ;
#14028=EDGE_CURVE ( 'NONE', #9252, #22886, #23511, .T. ) ;
#14075=VERTEX_POINT ( 'NONE', #7839 ) ;
#14090=ORIENTED_EDGE ( 'NONE', *, *, #8320, .F. ) ;
#14095=DIRECTION ( 'NONE',  ( -2.602084704489999637E-17, 1.000000000000000000, 0.000000000000000000 ) ) ;
#14096=CARTESIAN_POINT ( 'NONE',  ( -32.50000000000000000, 28.00000000000000000, -146.5552959529999839 ) ) ;
#14155=ORIENTED_EDGE ( 'NONE', *, *, #13601, .F. ) ;
#14166=VECTOR ( 'NONE', #9758, 1000.000000000000000 ) ;
#14169=CARTESIAN_POINT ( 'NONE',  ( -32.50000000000000000, -62.58229784560000297, -140.5449657050000098 ) ) ;
#14194=ADVANCED_FACE ( 'NONE', ( #4517 ), #13912, .F. ) ;
#14250=AXIS2_PLACEMENT_3D ( 'NONE', #10396, #17670, #8605 ) ;
#14293=DIRECTION ( 'NONE',  ( 0.000000000000000000, 1.000000000000000000, 0.000000000000000000 ) ) ;
#14302=DIRECTION ( 'NONE',  ( 0.000000000000000000, 1.000000000000000000, 0.000000000000000000 ) ) ;
#14400=CARTESIAN_POINT ( 'NONE',  ( -34.50000000000000000, 37.00000000000000000, -150.5552959529999839 ) ) ;
#14444=AXIS2_PLACEMENT_3D ( 'NONE', #18071, #9127, #16406 ) ;
#14491=DIRECTION ( 'NONE',  ( 0.7071067811866730279, 0.3390050494208429743, 0.6205445805637129775 ) ) ;
#14508=PLANE ( 'NONE',  #14444 ) ;
#14517=VERTEX_POINT ( 'NONE', #11492 ) ;
#14707=CARTESIAN_POINT ( 'NONE',  ( -32.50000000000000000, 28.00000000000000000, -144.0552959529999839 ) ) ;
#14714=LINE ( 'NONE', #21982, #17451 ) ;
#14757=LINE ( 'NONE', #2282, #3415 ) ;
#14809=APPLICATION_CONTEXT ( 'automotive_design' ) ;
#14826=ORIENTED_EDGE ( 'NONE', *, *, #15525, .T. ) ;
#14829=VECTOR ( 'NONE', #20408, 1000.000000000000000 ) ;
#14871=ORIENTED_EDGE ( 'NONE', *, *, #21121, .F. ) ;
#14872=DIRECTION ( 'NONE',  ( 0.000000000000000000, -1.000000000000000000, 0.000000000000000000 ) ) ;
#14912=AXIS2_PLACEMENT_3D ( 'NONE', #4510, #8181, #10326 ) ;
#14945=DIRECTION ( 'NONE',  ( 1.000000000000000000, 0.000000000000000000, 0.000000000000000000 ) ) ;
#14946=ORIENTED_EDGE ( 'NONE', *, *, #16018, .T. ) ;
#14997=EDGE_CURVE ( 'NONE', #6301, #22167, #12116, .T. ) ;
#15065=ORIENTED_EDGE ( 'NONE', *, *, #12652, .T. ) ;
#15081=LINE ( 'NONE', #6036, #7553 ) ;
#15101=ORIENTED_EDGE ( 'NONE', *, *, #19045, .F. ) ;
#15121=LINE ( 'NONE', #11422, #10454 ) ;
#15125=PLANE ( 'NONE',  #9923 ) ;
#15128=AXIS2_PLACEMENT_3D ( 'NONE', #2576, #15411, #22670 ) ;
#15168=EDGE_CURVE ( 'NONE', #14075, #6228, #4395, .T. ) ;
#15207=FACE_OUTER_BOUND ( 'NONE', #18005, .T. ) ;
#15299=DIRECTION ( 'NONE',  ( -1.701177084980000217E-20, -4.426606872460000157E-37, -1.000000000000000000 ) ) ;
#15343=ORIENTED_EDGE ( 'NONE', *, *, #10505, .F. ) ;
#15370=LINE ( 'NONE', #626, #13359 ) ;
#15387=CARTESIAN_POINT ( 'NONE',  ( -34.50000000000000000, 26.00000000000000000, -141.5552959529999839 ) ) ;
#15411=DIRECTION ( 'NONE',  ( 1.000000000000000000, 2.004714280773594901E-17, -1.095180403012019938E-17 ) ) ;
#15418=ORIENTED_EDGE ( 'NONE', *, *, #23347, .T. ) ;
#15420=ADVANCED_FACE ( 'NONE', ( #13260 ), #2460, .F. ) ;
#15441=DIRECTION ( 'NONE',  ( -1.000000000000000000, 0.000000000000000000, 0.000000000000000000 ) ) ;
#15450=CARTESIAN_POINT ( 'NONE',  ( -33.50000000000000000, -1.000000000000000000, -140.0552959529999839 ) ) ;
#15455=DIRECTION ( 'NONE',  ( 0.000000000000000000, -0.4794255386042033384, -0.8775825618903726477 ) ) ;
#15462=VECTOR ( 'NONE', #12351, 1000.000000000000000 ) ;
#15488=DIRECTION ( 'NONE',  ( -1.701177084980000217E-20, -4.426606872460000157E-37, -1.000000000000000000 ) ) ;
#15500=CIRCLE ( 'NONE', #19290, 2.000000000000001776 ) ;
#15509=ORIENTED_EDGE ( 'NONE', *, *, #22479, .T. ) ;
#15522=FACE_OUTER_BOUND ( 'NONE', #20293, .T. ) ;
#15525=EDGE_CURVE ( 'NONE', #8011, #22948, #13890, .T. ) ;
#15532=VECTOR ( 'NONE', #2158, 1000.000000000000000 ) ;
#15538=VERTEX_POINT ( 'NONE', #21246 ) ;
#15550=VECTOR ( 'NONE', #23231, 1000.000000000000000 ) ;
#15567=ORIENTED_EDGE ( 'NONE', *, *, #18394, .T. ) ;
#15576=VECTOR ( 'NONE', #15441, 1000.000000000000000 ) ;
#15582=ORIENTED_EDGE ( 'NONE', *, *, #12324, .T. ) ;
#15602=DIRECTION ( 'NONE',  ( 0.7071067811866730279, -0.3390050494208429743, -0.6205445805637129775 ) ) ;
#15641=FACE_OUTER_BOUND ( 'NONE', #5384, .T. ) ;
#15643=AXIS2_PLACEMENT_3D ( 'NONE', #9747, #20264, #9524 ) ;
#15669=ORIENTED_EDGE ( 'NONE', *, *, #11384, .F. ) ;
#15671=EDGE_LOOP ( 'NONE', ( #3787, #8594, #21270, #11332 ) ) ;
#15741=FACE_OUTER_BOUND ( 'NONE', #5783, .T. ) ;
#15743=DIRECTION ( 'NONE',  ( 0.000000000000000000, 0.000000000000000000, -1.000000000000000000 ) ) ;
#15755=ORIENTED_EDGE ( 'NONE', *, *, #13561, .T. ) ;
#15772=ORIENTED_EDGE ( 'NONE', *, *, #9731, .F. ) ;
#15774=ORIENTED_EDGE ( 'NONE', *, *, #22460, .T. ) ;
#15795=CARTESIAN_POINT ( 'NONE',  ( -32.50000000000000000, 65.58229784559999587, -147.5656262009999864 ) ) ;
#15804=CARTESIAN_POINT ( 'NONE',  ( -34.50000000000000000, -64.50000000000000000, -144.0552959529999839 ) ) ;
#15848=DIRECTION ( 'NONE',  ( -1.000000000000000000, -2.602084704489999637E-17, 1.701177084830000066E-20 ) ) ;
#15853=PLANE ( 'NONE',  #19601 ) ;
#15894=DIRECTION ( 'NONE',  ( 0.000000000000000000, -1.000000000000000000, 0.000000000000000000 ) ) ;
#15902=DIRECTION ( 'NONE',  ( 1.000000000000000000, 2.602084704489999637E-17, -1.701177084830000066E-20 ) ) ;
#16018=EDGE_CURVE ( 'NONE', #7005, #18905, #8575, .T. ) ;
#16036=ORIENTED_EDGE ( 'NONE', *, *, #20750, .F. ) ;
#16043=PLANE ( 'NONE',  #16723 ) ;
#16155=AXIS2_PLACEMENT_3D ( 'NONE', #13124, #7653, #12662 ) ;
#16157=EDGE_CURVE ( 'NONE', #1069, #14517, #7280, .T. ) ;
#16248=VERTEX_POINT ( 'NONE', #4403 ) ;
#16289=AXIS2_PLACEMENT_3D ( 'NONE', #13939, #15488, #19298 ) ;
#16321=VERTEX_POINT ( 'NONE', #17137 ) ;
#16366=VERTEX_POINT ( 'NONE', #21423 ) ;
#16370=CARTESIAN_POINT ( 'NONE',  ( -32.50000000000000000, 12.08229784559999942, -147.5656262009999864 ) ) ;
#16397=ORIENTED_EDGE ( 'NONE', *, *, #9731, .T. ) ;
#16400=DIRECTION ( 'NONE',  ( 2.602084704489999637E-17, -1.000000000000000000, -4.426606872070000353E-37 ) ) ;
#16406=DIRECTION ( 'NONE',  ( 0.000000000000000000, 4.426606872070000353E-37, -1.000000000000000000 ) ) ;
#16409=ORIENTED_EDGE ( 'NONE', *, *, #13561, .F. ) ;
#16422=LINE ( 'NONE', #7374, #19995 ) ;
#16424=DIRECTION ( 'NONE',  ( 0.000000000000000000, 0.000000000000000000, 1.000000000000000000 ) ) ;
#16440=FACE_OUTER_BOUND ( 'NONE', #2925, .T. ) ;
#16454=EDGE_CURVE ( 'NONE', #7907, #15538, #21307, .T. ) ;
#16546=CARTESIAN_POINT ( 'NONE',  ( -34.50000000000000000, 0.9999999999959999775, -144.0552959529999839 ) ) ;
#16602=DIRECTION ( 'NONE',  ( 0.000000000000000000, 1.000000000000000000, 0.000000000000000000 ) ) ;
#16627=EDGE_CURVE ( 'NONE', #10172, #19035, #19579, .T. ) ;
#16639=DIRECTION ( 'NONE',  ( -1.000000000000000000, 0.000000000000000000, 1.701177084980000217E-20 ) ) ;
#16641=SHAPE_REPRESENTATION ( 'Faceplate Support', ( #5025 ), #3536 ) ;
#16698=DIRECTION ( 'NONE',  ( 0.000000000000000000, -1.000000000000000000, 0.000000000000000000 ) ) ;
#16723=AXIS2_PLACEMENT_3D ( 'NONE', #5452, #16400, #9117 ) ;
#16726=LINE ( 'NONE', #20656, #13720 ) ;
#16727=ORIENTED_EDGE ( 'NONE', *, *, #16898, .F. ) ;
#16737=EDGE_LOOP ( 'NONE', ( #8306, #5194, #6367, #23228 ) ) ;
#16769=SURFACE_STYLE_USAGE ( .BOTH. , #6061 ) ;
#16781=EDGE_CURVE ( 'NONE', #22145, #941, #18425, .T. ) ;
#16789=EDGE_CURVE ( 'NONE', #5687, #1422, #9421, .T. ) ;
#16800=EDGE_CURVE ( 'NONE', #22948, #8011, #20335, .T. ) ;
#16802=CARTESIAN_POINT ( 'NONE',  ( -32.50000000000000000, 76.00000000000000000, -144.0552959529999839 ) ) ;
#16823=DIRECTION ( 'NONE',  ( 0.000000000000000000, 1.000000000000000000, 0.000000000000000000 ) ) ;
#16825=LINE ( 'NONE', #180, #10161 ) ;
#16866=CARTESIAN_POINT ( 'NONE',  ( -32.50000000000000000, -18.00000000000000000, -140.0552959529999839 ) ) ;
#16896=VERTEX_POINT ( 'NONE', #21953 ) ;
#16898=EDGE_CURVE ( 'NONE', #22304, #12661, #292, .T. ) ;
#16927=CARTESIAN_POINT ( 'NONE',  ( -32.50000000000000000, -74.00000000000000000, -155.5552959529999839 ) ) ;
#16952=EDGE_CURVE ( 'NONE', #5601, #3284, #6462, .T. ) ;
#16967=VERTEX_POINT ( 'NONE', #11678 ) ;
#16983=VERTEX_POINT ( 'NONE', #15387 ) ;
#16992=ORIENTED_EDGE ( 'NONE', *, *, #16157, .T. ) ;
#17022=CARTESIAN_POINT ( 'NONE',  ( -34.50000000000000000, 76.00000000000000000, -155.5552959529999839 ) ) ;
#17056=CARTESIAN_POINT ( 'NONE',  ( -34.50000000000000000, -74.00000000000000000, -132.5552959530000123 ) ) ;
#17062=DIRECTION ( 'NONE',  ( 1.000000000000000000, 2.004714280773594901E-17, -1.095180403012019938E-17 ) ) ;
#17084=DIRECTION ( 'NONE',  ( 0.000000000000000000, 0.000000000000000000, 1.000000000000000000 ) ) ;
#17095=VECTOR ( 'NONE', #1262, 1000.000000000000000 ) ;
#17113=VECTOR ( 'NONE', #13691, 1000.000000000000000 ) ;
#17115=EDGE_LOOP ( 'NONE', ( #17352, #14871, #13506, #3182 ) ) ;
#17128=DIRECTION ( 'NONE',  ( 1.000000000000000000, 2.004714280773594901E-17, -1.095180403012019938E-17 ) ) ;
#17137=CARTESIAN_POINT ( 'NONE',  ( -32.50000000000000000, 48.00000000000000000, -137.5552959530000123 ) ) ;
#17172=ADVANCED_FACE ( 'NONE', ( #15741 ), #15853, .F. ) ;
#17199=LINE ( 'NONE', #11591, #94 ) ;
#17207=FACE_OUTER_BOUND ( 'NONE', #7613, .T. ) ;
#17224=LINE ( 'NONE', #2955, #13201 ) ;
#17248=DIRECTION ( 'NONE',  ( 1.000000000000000000, 0.000000000000000000, -1.701177084980000217E-20 ) ) ;
#17274=EDGE_LOOP ( 'NONE', ( #14826, #19413, #2076, #20951 ) ) ;
#17288=VECTOR ( 'NONE', #5867, 1000.000000000000000 ) ;
#17328=EDGE_CURVE ( 'NONE', #12661, #14517, #15121, .T. ) ;
#17352=ORIENTED_EDGE ( 'NONE', *, *, #7784, .T. ) ;
#17366=AXIS2_PLACEMENT_3D ( 'NONE', #18115, #1951, #3482 ) ;
#17436=CARTESIAN_POINT ( 'NONE',  ( -34.50000000000000000, -74.00000000000000000, -132.5552959530000123 ) ) ;
#17451=VECTOR ( 'NONE', #5902, 1000.000000000000114 ) ;
#17494=PRESENTATION_STYLE_ASSIGNMENT (( #4651 ) ) ;
#17513=ORIENTED_EDGE ( 'NONE', *, *, #22575, .T. ) ;
#17549=EDGE_CURVE ( 'NONE', #13154, #76, #6660, .T. ) ;
#17551=EDGE_CURVE ( 'NONE', #1422, #3284, #16422, .T. ) ;
#17558=DIRECTION ( 'NONE',  ( 0.000000000000000000, 0.000000000000000000, 1.000000000000000000 ) ) ;
#17604=ORIENTED_EDGE ( 'NONE', *, *, #3978, .F. ) ;
#17633=CARTESIAN_POINT ( 'NONE',  ( -32.50000000000000000, -1.000000000000000000, -140.0552959529999839 ) ) ;
#17659=CARTESIAN_POINT ( 'NONE',  ( -32.50000000000000000, 14.00000000000000000, -144.0552959529999839 ) ) ;
#17670=DIRECTION ( 'NONE',  ( -1.000000000000000000, -2.602084704489999637E-17, 1.701177084830000066E-20 ) ) ;
#17697=ORIENTED_EDGE ( 'NONE', *, *, #4756, .T. ) ;
#17709=ORIENTED_EDGE ( 'NONE', *, *, #8210, .T. ) ;
#17716=VECTOR ( 'NONE', #10365, 1000.000000000000000 ) ;
#17775=AXIS2_PLACEMENT_3D ( 'NONE', #9713, #7373, #16639 ) ;
#17834=FACE_OUTER_BOUND ( 'NONE', #10596, .T. ) ;
#17850=ORIENTED_EDGE ( 'NONE', *, *, #17328, .T. ) ;
#17935=VECTOR ( 'NONE', #22476, 1000.000000000000000 ) ;
#17945=CARTESIAN_POINT ( 'NONE',  ( -32.50000000000000000, 46.00000000000000000, -146.5552959529999839 ) ) ;
#17991=FACE_BOUND ( 'NONE', #1638, .T. ) ;
#18005=EDGE_LOOP ( 'NONE', ( #3388, #14155, #21955, #19657 ) ) ;
#18071=CARTESIAN_POINT ( 'NONE',  ( -32.50000000000000000, -35.00000000000000000, -151.0552959529999839 ) ) ;
#18080=EDGE_CURVE ( 'NONE', #941, #22145, #11625, .T. ) ;
#18109=ADVANCED_FACE ( 'NONE', ( #5446 ), #21760, .F. ) ;
#18115=CARTESIAN_POINT ( 'NONE',  ( -34.50000000000000000, 67.50000000000000000, -144.0552959529999839 ) ) ;
#18148=ORIENTED_EDGE ( 'NONE', *, *, #16157, .F. ) ;
#18199=CARTESIAN_POINT ( 'NONE',  ( -34.50000000000000000, 48.00000000000000000, -146.5552959529999839 ) ) ;
#18220=ORIENTED_EDGE ( 'NONE', *, *, #21785, .F. ) ;
#18250=ADVANCED_FACE ( 'NONE', ( #15522 ), #23259, .F. ) ;
#18289=EDGE_LOOP ( 'NONE', ( #15567, #11956, #17513, #16397 ) ) ;
#18374=CARTESIAN_POINT ( 'NONE',  ( -32.50000000000000000, 37.00000000000000000, -150.5552959529999839 ) ) ;
#18379=VECTOR ( 'NONE', #11112, 1000.000000000000000 ) ;
#18394=EDGE_CURVE ( 'NONE', #16983, #18478, #1849, .T. ) ;
#18425=CIRCLE ( 'NONE', #14250, 2.000000000000000000 ) ;
#18442=DIRECTION ( 'NONE',  ( 0.7071067811866730279, 0.3390050494208429743, 0.6205445805637129775 ) ) ;
#18467=CARTESIAN_POINT ( 'NONE',  ( -34.50000000000000000, 76.00000000000000000, -132.5552959530000123 ) ) ;
#18478=VERTEX_POINT ( 'NONE', #11526 ) ;
#18552=( NAMED_UNIT ( * ) SI_UNIT ( $, .STERADIAN. ) SOLID_ANGLE_UNIT ( ) );
#18556=ORIENTED_EDGE ( 'NONE', *, *, #1419, .F. ) ;
#18557=LINE ( 'NONE', #4391, #15532 ) ;
#18565=LINE ( 'NONE', #9507, #10946 ) ;
#18566=ORIENTED_EDGE ( 'NONE', *, *, #4121, .T. ) ;
#18575=SURFACE_SIDE_STYLE ('',( #4064 ) ) ;
#18579=DIRECTION ( 'NONE',  ( 1.000000000000000000, 0.000000000000000000, -1.701177084980000217E-20 ) ) ;
#18624=LINE ( 'NONE', #13028, #14829 ) ;
#18647=VECTOR ( 'NONE', #4456, 1000.000000000000000 ) ;
#18657=CARTESIAN_POINT ( 'NONE',  ( -32.50000000000000000, 26.00000000000000000, -137.5552959530000123 ) ) ;
#18680=SHAPE_REPRESENTATION_RELATIONSHIP ( 'NONE' , 'NONE' ,  #16641, #5808 ) ;
#18685=DIRECTION ( 'NONE',  ( -1.000000000000000000, 0.000000000000000000, 0.000000000000000000 ) ) ;
#18711=EDGE_CURVE ( 'NONE', #15538, #9295, #9012, .T. ) ;
#18723=VECTOR ( 'NONE', #18685, 1000.000000000000000 ) ;
#18751=ORIENTED_EDGE ( 'NONE', *, *, #21337, .T. ) ;
#18762=ORIENTED_EDGE ( 'NONE', *, *, #19643, .F. ) ;
#18781=PLANE ( 'NONE',  #17775 ) ;
#18814=DIRECTION ( 'NONE',  ( 2.602084704489999637E-17, -1.000000000000000000, -4.426606872070000353E-37 ) ) ;
#18821=CARTESIAN_POINT ( 'NONE',  ( -34.50000000000000000, 76.00000000000000000, -144.0552959529999839 ) ) ;
#18850=ORIENTED_EDGE ( 'NONE', *, *, #6937, .T. ) ;
#18865=FACE_OUTER_BOUND ( 'NONE', #17274, .T. ) ;
#18883=DIRECTION ( 'NONE',  ( 0.000000000000000000, 0.000000000000000000, -1.000000000000000000 ) ) ;
#18905=VERTEX_POINT ( 'NONE', #18199 ) ;
#18939=CARTESIAN_POINT ( 'NONE',  ( -33.50000000000000000, 48.00000000000000000, -137.5552959530000123 ) ) ;
#18945=DIRECTION ( 'NONE',  ( 0.000000000000000000, 0.000000000000000000, 1.000000000000000000 ) ) ;
#18991=VERTEX_POINT ( 'NONE', #8386 ) ;
#19007=ORIENTED_EDGE ( 'NONE', *, *, #3029, .T. ) ;
#19025=ORIENTED_EDGE ( 'NONE', *, *, #22575, .F. ) ;
#19035=VERTEX_POINT ( 'NONE', #10035 ) ;
#19042=LINE ( 'NONE', #13920, #2654 ) ;
#19045=EDGE_CURVE ( 'NONE', #5687, #5601, #1026, .T. ) ;
#19137=LINE ( 'NONE', #10193, #17935 ) ;
#19148=CARTESIAN_POINT ( 'NONE',  ( -32.50000000000000000, 26.00000000000000000, -141.5552959529999839 ) ) ;
#19180=EDGE_CURVE ( 'NONE', #947, #76, #5524, .T. ) ;
#19199=CARTESIAN_POINT ( 'NONE',  ( -34.50000000000000000, 14.00000000000000000, -144.0552959529999839 ) ) ;
#19249=FACE_OUTER_BOUND ( 'NONE', #20336, .T. ) ;
#19275=CARTESIAN_POINT ( 'NONE',  ( -32.50000000000000000, 47.00000000000000000, -141.5552959529999839 ) ) ;
#19286=VECTOR ( 'NONE', #19307, 1000.000000000000000 ) ;
#19290=AXIS2_PLACEMENT_3D ( 'NONE', #10099, #969, #3106 ) ;
#19295=ORIENTED_EDGE ( 'NONE', *, *, #12083, .F. ) ;
#19298=DIRECTION ( 'NONE',  ( -1.000000000000000000, 0.000000000000000000, 1.701177084980000217E-20 ) ) ;
#19307=DIRECTION ( 'NONE',  ( 0.000000000000000000, 0.000000000000000000, -1.000000000000000000 ) ) ;
#19372=CARTESIAN_POINT ( 'NONE',  ( -34.50000000000000000, 76.00000000000000000, -132.5552959530000123 ) ) ;
#19413=ORIENTED_EDGE ( 'NONE', *, *, #2109, .F. ) ;
#19430=ADVANCED_FACE ( 'NONE', ( #19905 ), #21564, .F. ) ;
#19516=CONICAL_SURFACE ( 'NONE', #6422, 1.999999999999992450, 0.7853981633970000820 ) ;
#19519=CARTESIAN_POINT ( 'NONE',  ( -34.50000000000000000, 47.00000000000000000, -141.5552959529999839 ) ) ;
#19572=FACE_OUTER_BOUND ( 'NONE', #20079, .T. ) ;
#19579=LINE ( 'NONE', #23147, #11191 ) ;
#19584=MANIFOLD_SOLID_BREP ( 'lock_assembly.1\\lock body face plate inner.1\\PartBody', #7286 ) ;
#19601=AXIS2_PLACEMENT_3D ( 'NONE', #12278, #23002, #4916 ) ;
#19643=EDGE_CURVE ( 'NONE', #16248, #22660, #15500, .T. ) ;
#19657=ORIENTED_EDGE ( 'NONE', *, *, #12977, .T. ) ;
#19667=ORIENTED_EDGE ( 'NONE', *, *, #15168, .F. ) ;
#19732=ORIENTED_EDGE ( 'NONE', *, *, #19813, .T. ) ;
#19759=ORIENTED_EDGE ( 'NONE', *, *, #7611, .F. ) ;
#19769=DIRECTION ( 'NONE',  ( -1.000000000000000000, -2.602084704489999637E-17, 1.701177084830000066E-20 ) ) ;
#19799=VERTEX_POINT ( 'NONE', #20342 ) ;
#19813=EDGE_CURVE ( 'NONE', #11004, #18991, #9604, .T. ) ;
#19824=CARTESIAN_POINT ( 'NONE',  ( -33.50000000000000000, 46.00000000000000000, -141.5552959529999839 ) ) ;
#19870=ADVANCED_FACE ( 'NONE', ( #11502 ), #18781, .F. ) ;
#19905=FACE_OUTER_BOUND ( 'NONE', #23409, .T. ) ;
#19955=EDGE_LOOP ( 'NONE', ( #22959, #15772, #15065, #22991 ) ) ;
#19990=EDGE_CURVE ( 'NONE', #947, #13431, #17224, .T. ) ;
#19995=VECTOR ( 'NONE', #132, 1000.000000000000000 ) ;
#20004=CARTESIAN_POINT ( 'NONE',  ( -32.50000000000000000, 76.00000000000000000, -155.5552959529999839 ) ) ;
#20015=DIRECTION ( 'NONE',  ( 0.000000000000000000, -1.000000000000000000, 0.000000000000000000 ) ) ;
#20022=EDGE_CURVE ( 'NONE', #22145, #22886, #2728, .T. ) ;
#20040=CARTESIAN_POINT ( 'NONE',  ( -34.50000000000000000, 26.00000000000000000, -139.5552959529999839 ) ) ;
#20074=DIRECTION ( 'NONE',  ( 0.000000000000000000, 0.000000000000000000, -1.000000000000000000 ) ) ;
#20079=EDGE_LOOP ( 'NONE', ( #21978, #16992, #21180, #5922 ) ) ;
#20095=ORIENTED_EDGE ( 'NONE', *, *, #22316, .T. ) ;
#20107=DIRECTION ( 'NONE',  ( 0.000000000000000000, 0.000000000000000000, -1.000000000000000000 ) ) ;
#20147=DIRECTION ( 'NONE',  ( 0.000000000000000000, 1.000000000000000000, 0.000000000000000000 ) ) ;
#20160=ORIENTED_EDGE ( 'NONE', *, *, #16627, .T. ) ;
#20176=LINE ( 'NONE', #12895, #3338 ) ;
#20208=ORIENTED_EDGE ( 'NONE', *, *, #12652, .F. ) ;
#20224=AXIS2_PLACEMENT_3D ( 'NONE', #18467, #13344, #11433 ) ;
#20235=CARTESIAN_POINT ( 'NONE',  ( -32.50000000000000000, 37.00000000000000000, -137.5552959530000123 ) ) ;
#20264=DIRECTION ( 'NONE',  ( -2.602084704489999637E-17, 1.000000000000000000, 4.426606872070000353E-37 ) ) ;
#20271=EDGE_LOOP ( 'NONE', ( #18850, #11731, #10433, #2132 ) ) ;
#20293=EDGE_LOOP ( 'NONE', ( #22958, #10076, #20095, #22920 ) ) ;
#20323=SHAPE_DEFINITION_REPRESENTATION ( #8812, #16641 ) ;
#20329=LINE ( 'NONE', #22224, #6780 ) ;
#20335=CIRCLE ( 'NONE', #16155, 4.000000000000003553 ) ;
#20336=EDGE_LOOP ( 'NONE', ( #13757, #6382, #8615, #7824 ) ) ;
#20342=CARTESIAN_POINT ( 'NONE',  ( -32.50000000000000000, 26.00000000000000000, -150.5552959529999839 ) ) ;
#20343=ORIENTED_EDGE ( 'NONE', *, *, #18711, .F. ) ;
#20344=DIRECTION ( 'NONE',  ( -1.000000000000000000, 0.000000000000000000, 0.000000000000000000 ) ) ;
#20352=LINE ( 'NONE', #11401, #4198 ) ;
#20368=FILL_AREA_STYLE ('',( #385 ) ) ;
#20400=ADVANCED_FACE ( 'NONE', ( #18865 ), #317, .F. ) ;
#20408=DIRECTION ( 'NONE',  ( -1.000000000000000000, 0.000000000000000000, 0.000000000000000000 ) ) ;
#20416=DIRECTION ( 'NONE',  ( -1.000000000000000000, -2.602084704489999637E-17, 1.701177084830000066E-20 ) ) ;
#20443=PLANE ( 'NONE',  #7173 ) ;
#20491=AXIS2_PLACEMENT_3D ( 'NONE', #23078, #13804, #17248 ) ;
#20513=DIRECTION ( 'NONE',  ( 0.000000000000000000, 1.000000000000000000, 0.000000000000000000 ) ) ;
#20543=ADVANCED_FACE ( 'NONE', ( #6089 ), #623, .F. ) ;
#20612=FACE_OUTER_BOUND ( 'NONE', #20271, .T. ) ;
#20625=CONICAL_SURFACE ( 'NONE', #14912, 1.999999999999995115, 0.7853981633970000820 ) ;
#20656=CARTESIAN_POINT ( 'NONE',  ( -34.50000000000000000, 46.00000000000000000, -144.0552959529999839 ) ) ;
#20707=ORIENTED_EDGE ( 'NONE', *, *, #5153, .F. ) ;
#20709=EDGE_CURVE ( 'NONE', #941, #9252, #10106, .T. ) ;
#20750=EDGE_CURVE ( 'NONE', #5196, #10172, #12609, .T. ) ;
#20832=ORIENTED_EDGE ( 'NONE', *, *, #10591, .F. ) ;
#20951=ORIENTED_EDGE ( 'NONE', *, *, #7070, .T. ) ;
#21001=ORIENTED_EDGE ( 'NONE', *, *, #5153, .T. ) ;
#21049=ADVANCED_FACE ( 'NONE', ( #19249 ), #19516, .F. ) ;
#21076=LINE ( 'NONE', #19275, #1527 ) ;
#21078=( LENGTH_UNIT ( ) NAMED_UNIT ( * ) SI_UNIT ( .MILLI., .METRE. ) );
#21119=DIRECTION ( 'NONE',  ( 0.000000000000000000, 1.000000000000000000, 0.000000000000000000 ) ) ;
#21120=VECTOR ( 'NONE', #16823, 1000.000000000000000 ) ;
#21121=EDGE_CURVE ( 'NONE', #14075, #6301, #14714, .T. ) ;
#21136=VECTOR ( 'NONE', #20015, 1000.000000000000000 ) ;
#21180=ORIENTED_EDGE ( 'NONE', *, *, #4173, .T. ) ;
#21197=CARTESIAN_POINT ( 'NONE',  ( -33.50000000000000000, 26.00000000000000000, -146.5552959529999839 ) ) ;
#21246=CARTESIAN_POINT ( 'NONE',  ( -34.50000000000000000, 48.00000000000000000, -141.5552959529999839 ) ) ;
#21270=ORIENTED_EDGE ( 'NONE', *, *, #23514, .F. ) ;
#21303=ORIENTED_EDGE ( 'NONE', *, *, #1398, .T. ) ;
#21307=LINE ( 'NONE', #8194, #12730 ) ;
#21337=EDGE_CURVE ( 'NONE', #12661, #5687, #7279, .T. ) ;
#21339=CARTESIAN_POINT ( 'NONE',  ( -33.50000000000000000, 48.00000000000000000, -146.5552959529999839 ) ) ;
#21423=CARTESIAN_POINT ( 'NONE',  ( -34.50000000000000000, 46.00000000000000000, -146.5552959529999839 ) ) ;
#21470=ORIENTED_EDGE ( 'NONE', *, *, #8210, .F. ) ;
#21476=FACE_BOUND ( 'NONE', #6828, .T. ) ;
#21493=ORIENTED_EDGE ( 'NONE', *, *, #1770, .F. ) ;
#21511=CARTESIAN_POINT ( 'NONE',  ( -32.50000000000000000, 69.41770215440000413, -140.5449657050000098 ) ) ;
#21512=AXIS2_PLACEMENT_3D ( 'NONE', #5888, #20416, #16602 ) ;
#21564=CONICAL_SURFACE ( 'NONE', #17366, 1.999999999999992450, 0.7853981633970000820 ) ;
#21657=AXIS2_PLACEMENT_3D ( 'NONE', #2974, #17128, #15455 ) ;
#21677=VECTOR ( 'NONE', #14872, 1000.000000000000000 ) ;
#21730=EDGE_CURVE ( 'NONE', #18905, #5196, #19042, .T. ) ;
#21758=ORIENTED_EDGE ( 'NONE', *, *, #23514, .T. ) ;
#21760=PLANE ( 'NONE',  #1780 ) ;
#21785=EDGE_CURVE ( 'NONE', #2980, #7907, #21076, .T. ) ;
#21796=ORIENTED_EDGE ( 'NONE', *, *, #21730, .T. ) ;
#21947=VECTOR ( 'NONE', #20513, 1000.000000000000000 ) ;
#21953=CARTESIAN_POINT ( 'NONE',  ( -34.50000000000000000, 48.00000000000000000, -137.5552959530000123 ) ) ;
#21955=ORIENTED_EDGE ( 'NONE', *, *, #8152, .T. ) ;
#21956=ORIENTED_EDGE ( 'NONE', *, *, #16789, .F. ) ;
#21973=CIRCLE ( 'NONE', #11301, 4.000000000000003553 ) ;
#21978=ORIENTED_EDGE ( 'NONE', *, *, #11955, .T. ) ;
#21982=CARTESIAN_POINT ( 'NONE',  ( -33.42928932190000069, 68.97217712079999785, -141.3604938089999905 ) ) ;
#21998=LINE ( 'NONE', #16866, #11329 ) ;
#22093=DIRECTION ( 'NONE',  ( 0.000000000000000000, 0.000000000000000000, 1.000000000000000000 ) ) ;
#22129=EDGE_LOOP ( 'NONE', ( #8730, #19007, #11880, #6677 ) ) ;
#22145=VERTEX_POINT ( 'NONE', #4270 ) ;
#22167=VERTEX_POINT ( 'NONE', #15795 ) ;
#22181=CARTESIAN_POINT ( 'NONE',  ( -34.50000000000000000, 0.9999999999959999775, -155.5552959529999839 ) ) ;
#22212=ORIENTED_EDGE ( 'NONE', *, *, #10505, .T. ) ;
#22224=CARTESIAN_POINT ( 'NONE',  ( -34.50000000000000000, 37.00000000000000000, -137.5552959530000123 ) ) ;
#22240=LINE ( 'NONE', #20235, #21677 ) ;
#22246=( NAMED_UNIT ( * ) PLANE_ANGLE_UNIT ( ) SI_UNIT ( $, .RADIAN. ) );
#22253=LINE ( 'NONE', #5944, #18723 ) ;
#22271=DIRECTION ( 'NONE',  ( 0.000000000000000000, 4.426606872070000353E-37, -1.000000000000000000 ) ) ;
#22295=DIRECTION ( 'NONE',  ( 0.7071067811866730279, -0.3390050494208429743, -0.6205445805637129775 ) ) ;
#22304=VERTEX_POINT ( 'NONE', #19372 ) ;
#22316=EDGE_CURVE ( 'NONE', #16967, #73, #6864, .T. ) ;
#22328=VECTOR ( 'NONE', #20107, 1000.000000000000000 ) ;
#22362=( NAMED_UNIT ( * ) SI_UNIT ( $, .STERADIAN. ) SOLID_ANGLE_UNIT ( ) );
#22404=AXIS2_PLACEMENT_3D ( 'NONE', #6596, #15299, #22663 ) ;
#22424=DIRECTION ( 'NONE',  ( -1.701177084980000217E-20, -4.426606872460000157E-37, -1.000000000000000000 ) ) ;
#22426=ORIENTED_EDGE ( 'NONE', *, *, #5080, .T. ) ;
#22460=EDGE_CURVE ( 'NONE', #4685, #4452, #2227, .T. ) ;
#22476=DIRECTION ( 'NONE',  ( -1.000000000000000000, 0.000000000000000000, 0.000000000000000000 ) ) ;
#22479=EDGE_CURVE ( 'NONE', #9295, #16366, #16726, .T. ) ;
#22482=FILL_AREA_STYLE ('',( #2272 ) ) ;
#22527=CARTESIAN_POINT ( 'NONE',  ( -34.50000000000000000, -74.00000000000000000, -155.5552959529999839 ) ) ;
#22575=EDGE_CURVE ( 'NONE', #2789, #3632, #10372, .T. ) ;
#22632=LINE ( 'NONE', #18939, #14166 ) ;
#22657=ORIENTED_EDGE ( 'NONE', *, *, #5080, .F. ) ;
#22660=VERTEX_POINT ( 'NONE', #10836 ) ;
#22663=DIRECTION ( 'NONE',  ( -1.000000000000000000, 0.000000000000000000, 1.701177084980000217E-20 ) ) ;
#22670=DIRECTION ( 'NONE',  ( 0.000000000000000000, -0.4794255386042033384, -0.8775825618903726477 ) ) ;
#22684=DIRECTION ( 'NONE',  ( -1.000000000000000000, 0.000000000000000000, 0.000000000000000000 ) ) ;
#22746=ORIENTED_EDGE ( 'NONE', *, *, #16800, .F. ) ;
#22757=ADVANCED_FACE ( 'NONE', ( #5844 ), #15125, .F. ) ;
#22780=EDGE_LOOP ( 'NONE', ( #12847, #22657, #10085, #19759 ) ) ;
#22782=ADVANCED_FACE ( 'NONE', ( #20612 ), #9287, .F. ) ;
#22808=CARTESIAN_POINT ( 'NONE',  ( -32.50000000000000000, 46.00000000000000000, -141.5552959529999839 ) ) ;
#22857=DIRECTION ( 'NONE',  ( 0.000000000000000000, 0.000000000000000000, -1.000000000000000000 ) ) ;
#22859=( NAMED_UNIT ( * ) SI_UNIT ( $, .STERADIAN. ) SOLID_ANGLE_UNIT ( ) );
#22886=VERTEX_POINT ( 'NONE', #6551 ) ;
#22903=ORIENTED_EDGE ( 'NONE', *, *, #2191, .F. ) ;
#22905=DIRECTION ( 'NONE',  ( 1.701177084980000217E-20, 4.426606872460000157E-37, 1.000000000000000000 ) ) ;
#22920=ORIENTED_EDGE ( 'NONE', *, *, #8683, .T. ) ;
#22948=VERTEX_POINT ( 'NONE', #14169 ) ;
#22958=ORIENTED_EDGE ( 'NONE', *, *, #8320, .T. ) ;
#22959=ORIENTED_EDGE ( 'NONE', *, *, #11384, .T. ) ;
#22991=ORIENTED_EDGE ( 'NONE', *, *, #8408, .T. ) ;
#23002=DIRECTION ( 'NONE',  ( 1.701177084980000217E-20, 4.426606872460000157E-37, 1.000000000000000000 ) ) ;
#23078=CARTESIAN_POINT ( 'NONE',  ( -32.50000000000000000, 26.00000000000000000, -146.5552959529999839 ) ) ;
#23098=( GEOMETRIC_REPRESENTATION_CONTEXT ( 3 ) GLOBAL_UNCERTAINTY_ASSIGNED_CONTEXT ( ( #9203 ) ) GLOBAL_UNIT_ASSIGNED_CONTEXT ( ( #21078, #4764, #22859 ) ) REPRESENTATION_CONTEXT ( 'NONE', 'WORKASPACE' ) );
#23142=CARTESIAN_POINT ( 'NONE',  ( -33.50000000000000000, 28.00000000000000000, -146.5552959529999839 ) ) ;
#23147=CARTESIAN_POINT ( 'NONE',  ( -34.50000000000000000, 26.00000000000000000, -148.5552959529999839 ) ) ;
#23208=ADVANCED_FACE ( 'NONE', ( #2041 ), #11394, .F. ) ;
#23228=ORIENTED_EDGE ( 'NONE', *, *, #16454, .T. ) ;
#23230=ORIENTED_EDGE ( 'NONE', *, *, #14028, .F. ) ;
#23231=DIRECTION ( 'NONE',  ( 0.000000000000000000, 0.000000000000000000, -1.000000000000000000 ) ) ;
#23259=PLANE ( 'NONE',  #23421 ) ;
#23347=EDGE_CURVE ( 'NONE', #6863, #5196, #19137, .T. ) ;
#23350=CARTESIAN_POINT ( 'NONE',  ( -34.50000000000000000, -64.50000000000000000, -144.0552959529999839 ) ) ;
#23370=VERTEX_POINT ( 'NONE', #17945 ) ;
#23409=EDGE_LOOP ( 'NONE', ( #5068, #11629, #453, #11356 ) ) ;
#23421=AXIS2_PLACEMENT_3D ( 'NONE', #14096, #13858, #6950 ) ;
#23455=FACE_BOUND ( 'NONE', #15671, .T. ) ;
#23487=CARTESIAN_POINT ( 'NONE',  ( -32.50000000000000000, 0.9999999999959999775, -144.0552959529999839 ) ) ;
#23493=DIRECTION ( 'NONE',  ( -1.000000000000000000, 0.000000000000000000, 0.000000000000000000 ) ) ;
#23497=ORIENTED_EDGE ( 'NONE', *, *, #11837, .T. ) ;
#23503=VECTOR ( 'NONE', #15602, 1000.000000000000114 ) ;
#23511=CIRCLE ( 'NONE', #13237, 4.000000000000001776 ) ;
#23514=EDGE_CURVE ( 'NONE', #76, #11004, #17199, .T. ) ;
#23524=CARTESIAN_POINT ( 'NONE',  ( -34.50000000000000000, 66.54114892279999083, -145.8104610769999852 ) ) ;
#23531=DIRECTION ( 'NONE',  ( -1.000000000000000000, -2.602084704489999637E-17, 1.701177084830000066E-20 ) ) ;
ENDSEC;
END-ISO-10303-21;
